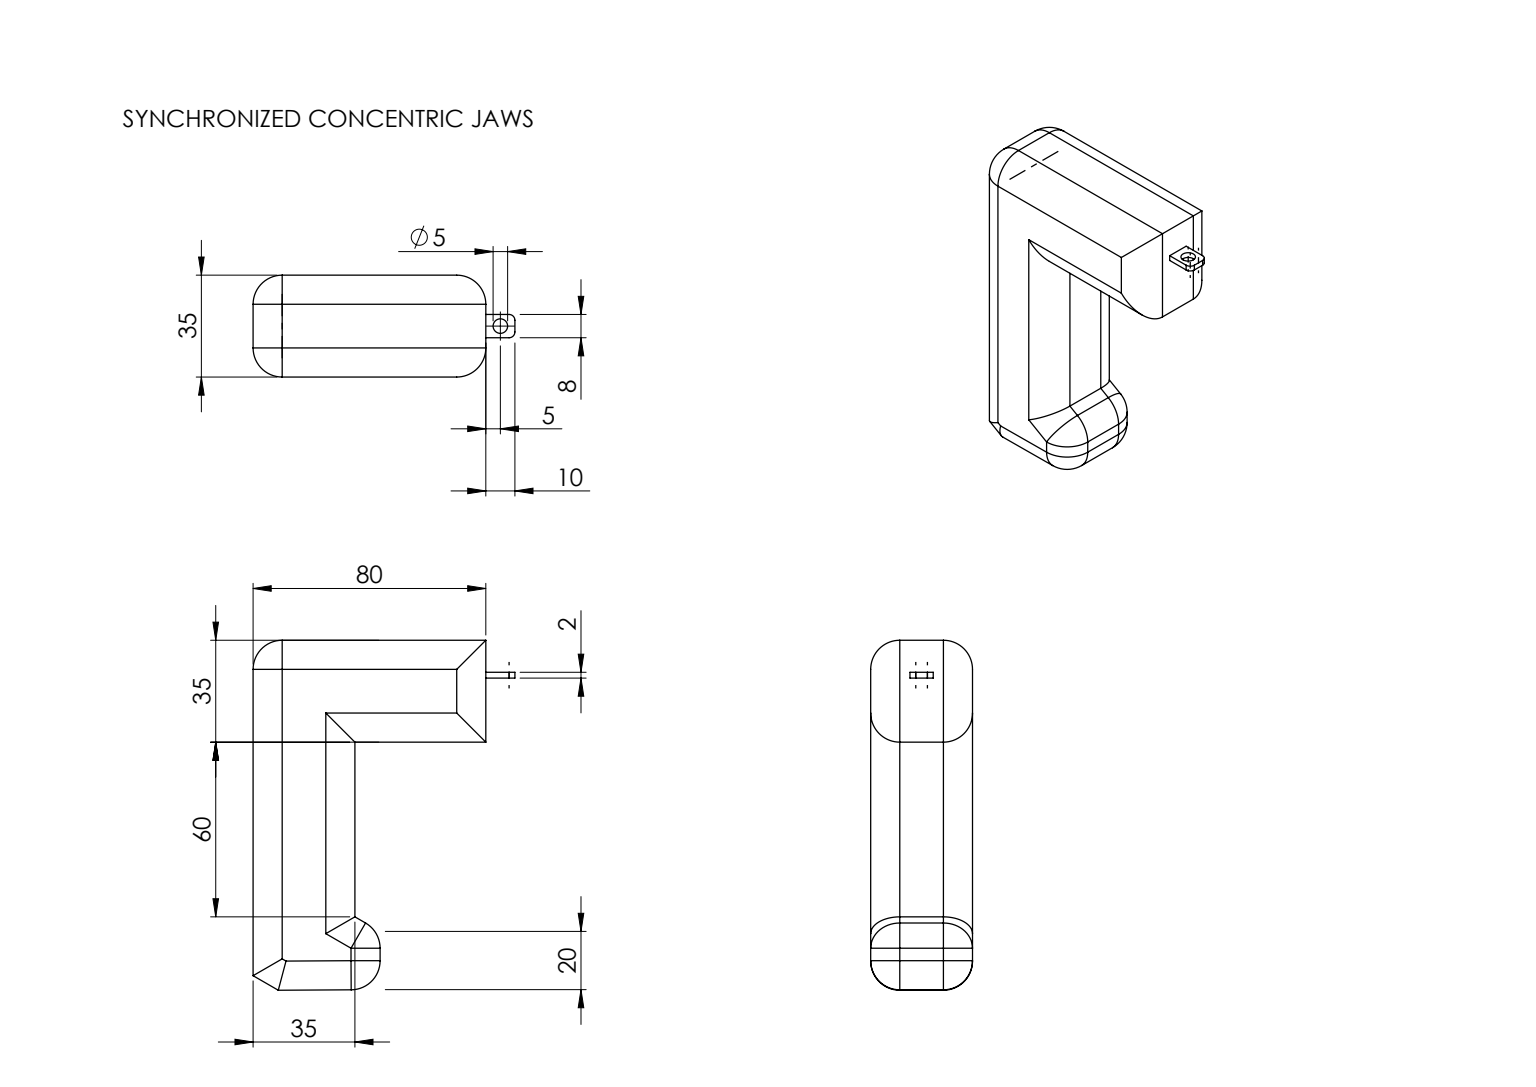
ISO-10303-21;
HEADER;
FILE_DESCRIPTION (('STEP AP214'),
    '1' );
FILE_NAME ('Synchronized Concentric Jaws.step',
    '2026-10-08T13:56:24',
    ( '' ),
    ( '' ),
    'SwSTEP 2.0',
    'SolidWorks 2026',
    '' );
FILE_SCHEMA (( 'AUTOMOTIVE_DESIGN' ));
ENDSEC;

DATA;
#2=EDGE_CURVE ( 'NONE', #5376, #11920, #8952, .T. ) ;
#20=ORIENTED_EDGE ( 'NONE', *, *, #13802, .F. ) ;
#26=ORIENTED_EDGE ( 'NONE', *, *, #11739, .T. ) ;
#47=FACE_OUTER_BOUND ( 'NONE', #13583, .T. ) ;
#72=ORIENTED_EDGE ( 'NONE', *, *, #13780, .T. ) ;
#78=DIRECTION ( 'NONE',  ( -1.000000000000000000, 0.000000000000000000, 0.000000000000000000 ) ) ;
#80=LINE ( 'NONE', #11141, #9950 ) ;
#112=DIRECTION ( 'NONE',  ( -1.925929944387236904E-30, 1.000000000000000000, -1.387778780781445676E-15 ) ) ;
#145=EDGE_CURVE ( 'NONE', #14420, #4422, #3824, .T. ) ;
#155=AXIS2_PLACEMENT_3D ( 'NONE', #3936, #13786, #7593 ) ;
#160=VECTOR ( 'NONE', #2348, 1000.000000000000000 ) ;
#188=EDGE_LOOP ( 'NONE', ( #9536, #20, #1499, #15874 ) ) ;
#190=VECTOR ( 'NONE', #3523, 1000.000000000000000 ) ;
#206=ORIENTED_EDGE ( 'NONE', *, *, #3407, .T. ) ;
#212=CARTESIAN_POINT ( 'NONE',  ( -44.99999999999999289, -11.00000000000000178, 4.000000000000831335 ) ) ;
#224=ORIENTED_EDGE ( 'NONE', *, *, #11721, .F. ) ;
#231=AXIS2_PLACEMENT_3D ( 'NONE', #4894, #14440, #11914 ) ;
#238=CARTESIAN_POINT ( 'NONE',  ( -115.0000000000000142, -3.122502256758252770E-14, 7.500000000000001776 ) ) ;
#253=CARTESIAN_POINT ( 'NONE',  ( -36.99999999999999289, -11.00000000000000178, 4.000000000000832223 ) ) ;
#283=ORIENTED_EDGE ( 'NONE', *, *, #4424, .F. ) ;
#306=ORIENTED_EDGE ( 'NONE', *, *, #14745, .F. ) ;
#310=DIRECTION ( 'NONE',  ( -1.000000000000000000, -2.775557561562892929E-15, 0.000000000000000000 ) ) ;
#317=FACE_OUTER_BOUND ( 'NONE', #13857, .T. ) ;
#319=CARTESIAN_POINT ( 'NONE',  ( -158.0560796608385488, -84.57531754730580076, 7.500000000000001776 ) ) ;
#326=ORIENTED_EDGE ( 'NONE', *, *, #10294, .F. ) ;
#344=ORIENTED_EDGE ( 'NONE', *, *, #14576, .T. ) ;
#350=CARTESIAN_POINT ( 'NONE',  ( -90.00000000000000000, -95.00000000000000000, 7.500000000000001776 ) ) ;
#373=ORIENTED_EDGE ( 'NONE', *, *, #7059, .F. ) ;
#393=EDGE_LOOP ( 'NONE', ( #15689, #8043, #13858, #8283 ) ) ;
#394=DIRECTION ( 'NONE',  ( -0.000000000000000000, -1.000000000000000000, -0.000000000000000000 ) ) ;
#396=SHAPE_REPRESENTATION ( 'Synchronized Concentric Jaws', ( #3223 ), #1155 ) ;
#443=ORIENTED_EDGE ( 'NONE', *, *, #6817, .F. ) ;
#451=ADVANCED_FACE ( 'NONE', ( #852 ), #7980, .T. ) ;
#461=ORIENTED_EDGE ( 'NONE', *, *, #7687, .F. ) ;
#466=AXIS2_PLACEMENT_3D ( 'NONE', #5707, #10643, #4493 ) ;
#472=DIRECTION ( 'NONE',  ( 0.000000000000000000, -1.000000000000000000, 0.000000000000000000 ) ) ;
#486=DIRECTION ( 'NONE',  ( -1.387778780781446464E-15, -1.000000000000000000, 1.387778780781447648E-15 ) ) ;
#525=( NAMED_UNIT ( * ) SI_UNIT ( $, .STERADIAN. ) SOLID_ANGLE_UNIT ( ) );
#546=ORIENTED_EDGE ( 'NONE', *, *, #11089, .F. ) ;
#549=FACE_OUTER_BOUND ( 'NONE', #2959, .T. ) ;
#554=FACE_OUTER_BOUND ( 'NONE', #8051, .T. ) ;
#559=LINE ( 'NONE', #10495, #3498 ) ;
#564=ORIENTED_EDGE ( 'NONE', *, *, #15075, .T. ) ;
#582=VECTOR ( 'NONE', #7048, 1000.000000000000000 ) ;
#586=EDGE_CURVE ( 'NONE', #13829, #5811, #14718, .T. ) ;
#597=DIRECTION ( 'NONE',  ( 1.000000000000000000, 1.239088197126290324E-16, -0.000000000000000000 ) ) ;
#617=CARTESIAN_POINT ( 'NONE',  ( -81.33974596215558961, -105.7735026918962404, 17.50000000000000000 ) ) ;
#619=EDGE_LOOP ( 'NONE', ( #15665, #842, #2905, #10808 ) ) ;
#630=CARTESIAN_POINT ( 'NONE',  ( -91.28042740779480368, -120.0589677227266918, -7.500000000000000000 ) ) ;
#645=AXIS2_PLACEMENT_3D ( 'NONE', #6232, #7360, #12268 ) ;
#651=LINE ( 'NONE', #15677, #14820 ) ;
#658=VERTEX_POINT ( 'NONE', #6156 ) ;
#665=CARTESIAN_POINT ( 'NONE',  ( -94.14213562373093680, -97.39146311738103634, 17.50000000000001421 ) ) ;
#677=VECTOR ( 'NONE', #5737, 1000.000000000000000 ) ;
#683=CARTESIAN_POINT ( 'NONE',  ( -44.99999999999999289, -35.00000000000000000, 17.50000000000000000 ) ) ;
#696=ORIENTED_EDGE ( 'NONE', *, *, #9480, .F. ) ;
#707=CARTESIAN_POINT ( 'NONE',  ( -99.99999999999998579, -25.00000000000000711, 17.50000000000000000 ) ) ;
#718=ORIENTED_EDGE ( 'NONE', *, *, #3664, .F. ) ;
#722=CYLINDRICAL_SURFACE ( 'NONE', #11218, 10.00000000000000000 ) ;
#757=VERTEX_POINT ( 'NONE', #7935 ) ;
#765=DIRECTION ( 'NONE',  ( -0.000000000000000000, -0.000000000000000000, -1.000000000000000000 ) ) ;
#770=EDGE_LOOP ( 'NONE', ( #1058, #1735, #5015, #1295 ) ) ;
#785=CARTESIAN_POINT ( 'NONE',  ( -114.9999999999999858, -115.2072594216369907, 17.50000000000000000 ) ) ;
#794=VERTEX_POINT ( 'NONE', #12509 ) ;
#798=DIRECTION ( 'NONE',  ( 0.4999999999999976685, 0.8660254037844399289, 0.000000000000000000 ) ) ;
#807=LINE ( 'NONE', #5727, #13340 ) ;
#811=DIRECTION ( 'NONE',  ( 1.319090325525611458E-16, 1.000000000000000000, 0.000000000000000000 ) ) ;
#820=CARTESIAN_POINT ( 'NONE',  ( -54.99999999999999289, -25.00000000000000000, 17.50000000000000000 ) ) ;
#842=ORIENTED_EDGE ( 'NONE', *, *, #8606, .F. ) ;
#845=LINE ( 'NONE', #15641, #3770 ) ;
#852=FACE_OUTER_BOUND ( 'NONE', #5733, .T. ) ;
#883=CARTESIAN_POINT ( 'NONE',  ( -39.99999999999999289, -11.00000000000000178, -2.500000000000079492 ) ) ;
#930=ORIENTED_EDGE ( 'NONE', *, *, #7501, .T. ) ;
#964=ORIENTED_EDGE ( 'NONE', *, *, #14576, .F. ) ;
#966=ORIENTED_EDGE ( 'NONE', *, *, #12050, .T. ) ;
#977=DIRECTION ( 'NONE',  ( -0.8660254037844401509, 0.4999999999999973355, -0.000000000000000000 ) ) ;
#979=EDGE_CURVE ( 'NONE', #13100, #8026, #12847, .T. ) ;
#992=ADVANCED_FACE ( 'NONE', ( #2100 ), #5909, .T. ) ;
#1013=CARTESIAN_POINT ( 'NONE',  ( -150.5560796608385203, -71.58493649053926333, -17.50000000000000000 ) ) ;
#1024=ORIENTED_EDGE ( 'NONE', *, *, #7059, .T. ) ;
#1028=FACE_BOUND ( 'NONE', #13834, .T. ) ;
#1046=DIRECTION ( 'NONE',  ( 0.9999824063907751803, 0.005931855436079011210, -0.000000000000000000 ) ) ;
#1058=ORIENTED_EDGE ( 'NONE', *, *, #12944, .T. ) ;
#1060=EDGE_CURVE ( 'NONE', #5100, #14039, #4611, .T. ) ;
#1072=EDGE_CURVE ( 'NONE', #12769, #13901, #14197, .T. ) ;
#1083=CARTESIAN_POINT ( 'NONE',  ( -111.3391301858327296, -111.5473609024183475, 17.50000000000000000 ) ) ;
#1090=CYLINDRICAL_SURFACE ( 'NONE', #14091, 10.00000000000000000 ) ;
#1114=EDGE_CURVE ( 'NONE', #794, #15817, #9839, .T. ) ;
#1117=ORIENTED_EDGE ( 'NONE', *, *, #12225, .T. ) ;
#1129=DIRECTION ( 'NONE',  ( 0.000000000000000000, -0.000000000000000000, -1.000000000000000000 ) ) ;
#1148=ORIENTED_EDGE ( 'NONE', *, *, #5739, .F. ) ;
#1155=( GEOMETRIC_REPRESENTATION_CONTEXT ( 3 ) GLOBAL_UNCERTAINTY_ASSIGNED_CONTEXT ( ( #5133 ) ) GLOBAL_UNIT_ASSIGNED_CONTEXT ( ( #12689, #7870, #525 ) ) REPRESENTATION_CONTEXT ( 'NONE', 'WORKASPACE' ) );
#1159=CARTESIAN_POINT ( 'NONE',  ( -113.6871902368262965, -110.1917077999038099, -17.50000000000000000 ) ) ;
#1170=EDGE_LOOP ( 'NONE', ( #3935, #2515, #6182 ) ) ;
#1175=AXIS2_PLACEMENT_3D ( 'NONE', #12176, #78, #12343 ) ;
#1181=EDGE_CURVE ( 'NONE', #6165, #13829, #13462, .T. ) ;
#1200=CARTESIAN_POINT ( 'NONE',  ( -81.33974596215560382, -110.0591436588189538, -7.500000000000000000 ) ) ;
#1203=DIRECTION ( 'NONE',  ( 1.000000000000000000, 0.000000000000000000, -0.000000000000000000 ) ) ;
#1226=FACE_OUTER_BOUND ( 'NONE', #7970, .T. ) ;
#1242=VECTOR ( 'NONE', #8938, 1000.000000000000000 ) ;
#1255=VECTOR ( 'NONE', #10833, 1000.000000000000000 ) ;
#1259=EDGE_CURVE ( 'NONE', #10280, #10210, #6230, .T. ) ;
#1261=EDGE_CURVE ( 'NONE', #11117, #5376, #7210, .T. ) ;
#1276=CARTESIAN_POINT ( 'NONE',  ( -55.00000000000000000, -1.734723475976807094E-15, 17.50000000000000000 ) ) ;
#1290=DIRECTION ( 'NONE',  ( 0.000000000000000000, 0.000000000000000000, -1.000000000000000000 ) ) ;
#1295=ORIENTED_EDGE ( 'NONE', *, *, #8606, .T. ) ;
#1306=DIRECTION ( 'NONE',  ( -0.8660254037844407060, 0.4999999999999965583, 0.000000000000000000 ) ) ;
#1314=ORIENTED_EDGE ( 'NONE', *, *, #10414, .F. ) ;
#1344=DIRECTION ( 'NONE',  ( 1.319090325525611458E-16, 1.000000000000000000, -0.000000000000000000 ) ) ;
#1352=DIRECTION ( 'NONE',  ( 0.000000000000000000, 1.000000000000000000, 0.000000000000000000 ) ) ;
#1360=DIRECTION ( 'NONE',  ( -0.000000000000000000, 0.000000000000000000, 1.000000000000000000 ) ) ;
#1362=FACE_OUTER_BOUND ( 'NONE', #8809, .T. ) ;
#1372=ORIENTED_EDGE ( 'NONE', *, *, #14448, .F. ) ;
#1395=AXIS2_PLACEMENT_3D ( 'NONE', #13554, #2487, #7448 ) ;
#1419=ADVANCED_FACE ( 'NONE', ( #7691 ), #1687, .F. ) ;
#1477=CYLINDRICAL_SURFACE ( 'NONE', #2817, 10.00000000000000000 ) ;
#1496=CARTESIAN_POINT ( 'NONE',  ( -49.14213562373093680, -4.142135623730950122, 17.49999999999999645 ) ) ;
#1498=DIRECTION ( 'NONE',  ( -1.000000000000000000, 1.387778780781446464E-15, 0.000000000000000000 ) ) ;
#1499=ORIENTED_EDGE ( 'NONE', *, *, #1640, .F. ) ;
#1500=DIRECTION ( 'NONE',  ( 1.982541115402065110E-16, -1.000000000000000000, 0.000000000000000000 ) ) ;
#1508=CARTESIAN_POINT ( 'NONE',  ( -91.33974596215558961, -110.0591436588189254, 7.500000000000001776 ) ) ;
#1515=FACE_OUTER_BOUND ( 'NONE', #7353, .T. ) ;
#1529=DIRECTION ( 'NONE',  ( -1.387778780781446464E-15, -1.000000000000000000, -0.000000000000000000 ) ) ;
#1530=EDGE_LOOP ( 'NONE', ( #4141, #4262 ) ) ;
#1541=LINE ( 'NONE', #13807, #12251 ) ;
#1545=ORIENTED_EDGE ( 'NONE', *, *, #13780, .F. ) ;
#1547=VERTEX_POINT ( 'NONE', #14221 ) ;
#1560=CARTESIAN_POINT ( 'NONE',  ( -114.4056415360013688, -110.1959696241292335, -17.50000000000000000 ) ) ;
#1570=CARTESIAN_POINT ( 'NONE',  ( -55.00000000000000000, -10.00000000000000178, 17.50000000000000000 ) ) ;
#1587=CARTESIAN_POINT ( 'NONE',  ( -44.99999999999999289, -11.00000000000000178, -3.999999999999170885 ) ) ;
#1589=CARTESIAN_POINT ( 'NONE',  ( -49.14213562373093680, -30.85786437626904899, -17.49999999999999645 ) ) ;
#1597=VERTEX_POINT ( 'NONE', #11053 ) ;
#1610=EDGE_CURVE ( 'NONE', #10210, #14193, #2463, .T. ) ;
#1614=ORIENTED_EDGE ( 'NONE', *, *, #11960, .F. ) ;
#1640=EDGE_CURVE ( 'NONE', #15020, #3371, #4274, .T. ) ;
#1649=CARTESIAN_POINT ( 'NONE',  ( -116.3391301858327296, -120.2076149402627294, 7.500000000000001776 ) ) ;
#1652=DIRECTION ( 'NONE',  ( 0.000000000000000000, 0.000000000000000000, 1.000000000000000000 ) ) ;
#1684=EDGE_CURVE ( 'NONE', #4500, #5972, #13528, .T. ) ;
#1687=CYLINDRICAL_SURFACE ( 'NONE', #11678, 2.500000000000909495 ) ;
#1702=ORIENTED_EDGE ( 'NONE', *, *, #2061, .F. ) ;
#1727=DIRECTION ( 'NONE',  ( -0.000000000000000000, -1.000000000000000000, -0.000000000000000000 ) ) ;
#1734=DIRECTION ( 'NONE',  ( -1.982541115402065110E-16, 1.000000000000000000, 0.000000000000000000 ) ) ;
#1735=ORIENTED_EDGE ( 'NONE', *, *, #4357, .T. ) ;
#1736=ORIENTED_EDGE ( 'NONE', *, *, #7501, .F. ) ;
#1743=CIRCLE ( 'NONE', #3807, 9.999999999999994671 ) ;
#1763=CARTESIAN_POINT ( 'NONE',  ( -91.33974596215560382, -110.0591436588189396, -17.50000000000000000 ) ) ;
#1815=ORIENTED_EDGE ( 'NONE', *, *, #11551, .T. ) ;
#1858=CARTESIAN_POINT ( 'NONE',  ( -89.99999999999997158, -95.00000000000001421, 13.35786437626905965 ) ) ;
#1884=CYLINDRICAL_SURFACE ( 'NONE', #12589, 2.000000000000000888 ) ;
#1886=VERTEX_POINT ( 'NONE', #9424 ) ;
#1893=DIRECTION ( 'NONE',  ( -0.000000000000000000, -1.000000000000000000, -0.000000000000000000 ) ) ;
#1905=( BOUNDED_CURVE ( )  B_SPLINE_CURVE ( 3, ( #6211, #13529, #3857, #9909 ),
 .UNSPECIFIED., .F., .F. ) 
 B_SPLINE_CURVE_WITH_KNOTS ( ( 4, 4 ),
 ( 1.570796326794895226, 3.141592653589793116 ),
 .UNSPECIFIED. ) 
 CURVE ( )  GEOMETRIC_REPRESENTATION_ITEM ( )  RATIONAL_B_SPLINE_CURVE ( ( 1.000000000000000000, 0.8047378541243646044, 0.8047378541243646044, 1.000000000000000000 ) ) 
 REPRESENTATION_ITEM ( '' )  );
#1936=ORIENTED_EDGE ( 'NONE', *, *, #15075, .F. ) ;
#1959=CARTESIAN_POINT ( 'NONE',  ( -115.0000000000000142, -10.00000000000000888, 7.500000000000001776 ) ) ;
#1995=EDGE_CURVE ( 'NONE', #14464, #5100, #13505, .T. ) ;
#2019=VECTOR ( 'NONE', #7235, 1000.000000000000000 ) ;
#2023=CARTESIAN_POINT ( 'NONE',  ( -45.00000000000000000, 0.000000000000000000, 17.50000000000000000 ) ) ;
#2033=VECTOR ( 'NONE', #10246, 1000.000000000000000 ) ;
#2042=EDGE_CURVE ( 'NONE', #15020, #15896, #12067, .T. ) ;
#2055=CARTESIAN_POINT ( 'NONE',  ( -114.4056415360013688, -110.1959696241292335, 7.500000000000001776 ) ) ;
#2058=DIRECTION ( 'NONE',  ( 0.000000000000000000, 0.000000000000000000, -1.000000000000000000 ) ) ;
#2060=CARTESIAN_POINT ( 'NONE',  ( -116.3391301858327296, -120.2076149402627294, -7.500000000000000000 ) ) ;
#2061=EDGE_CURVE ( 'NONE', #14193, #7180, #15739, .T. ) ;
#2066=LINE ( 'NONE', #785, #13594 ) ;
#2084=CARTESIAN_POINT ( 'NONE',  ( -114.9999999999999858, -109.4337567297407219, -17.50000000000000000 ) ) ;
#2099=CARTESIAN_POINT ( 'NONE',  ( -44.99999999999999289, -35.00000000000000000, 17.50000000000000000 ) ) ;
#2100=FACE_OUTER_BOUND ( 'NONE', #15094, .T. ) ;
#2125=ORIENTED_EDGE ( 'NONE', *, *, #10428, .T. ) ;
#2133=AXIS2_PLACEMENT_3D ( 'NONE', #13779, #2714, #472 ) ;
#2153=PRODUCT_DEFINITION ( 'UNKNOWN', '', #5085, #2371 ) ;
#2155=LINE ( 'NONE', #12005, #190 ) ;
#2212=DIRECTION ( 'NONE',  ( 0.000000000000000000, 1.000000000000000000, 0.000000000000000000 ) ) ;
#2224=CIRCLE ( 'NONE', #11263, 2.500000000000909495 ) ;
#2256=SPHERICAL_SURFACE ( 'NONE', #9506, 10.00000000000000000 ) ;
#2258=AXIS2_PLACEMENT_3D ( 'NONE', #10852, #15792, #7303 ) ;
#2293=EDGE_LOOP ( 'NONE', ( #12874, #3623, #1545, #4562 ) ) ;
#2308=AXIS2_PLACEMENT_3D ( 'NONE', #7872, #8843, #13748 ) ;
#2311=EDGE_LOOP ( 'NONE', ( #5185, #10664, #326, #13860 ) ) ;
#2314=CARTESIAN_POINT ( 'NONE',  ( -115.0000000000000142, -10.00000000000000888, 7.500000000000001776 ) ) ;
#2315=CARTESIAN_POINT ( 'NONE',  ( -114.9999999999999858, -109.4337567297407219, -17.50000000000000000 ) ) ;
#2327=ORIENTED_EDGE ( 'NONE', *, *, #13355, .F. ) ;
#2332=ORIENTED_EDGE ( 'NONE', *, *, #12839, .T. ) ;
#2334=EDGE_CURVE ( 'NONE', #3131, #15817, #13089, .T. ) ;
#2345=FACE_BOUND ( 'NONE', #1530, .T. ) ;
#2348=DIRECTION ( 'NONE',  ( -6.938893903907228378E-16, -1.000000000000000000, 0.000000000000000000 ) ) ;
#2370=DIRECTION ( 'NONE',  ( -1.982541115402065110E-16, 1.000000000000000000, 0.000000000000000000 ) ) ;
#2371=PRODUCT_DEFINITION_CONTEXT ( 'detailed design', #7449, 'design' ) ;
#2385=DIRECTION ( 'NONE',  ( 1.982541115402065110E-16, -1.000000000000000000, 0.000000000000000000 ) ) ;
#2396=ORIENTED_EDGE ( 'NONE', *, *, #12301, .F. ) ;
#2413=ORIENTED_EDGE ( 'NONE', *, *, #14745, .T. ) ;
#2414=EDGE_CURVE ( 'NONE', #13901, #3131, #8820, .T. ) ;
#2441=FACE_OUTER_BOUND ( 'NONE', #3474, .T. ) ;
#2442=CARTESIAN_POINT ( 'NONE',  ( -45.00000000000000000, 0.000000000000000000, -7.500000000000000000 ) ) ;
#2447=ADVANCED_FACE ( 'NONE', ( #4855 ), #9781, .T. ) ;
#2463=LINE ( 'NONE', #12241, #4705 ) ;
#2466=DIRECTION ( 'NONE',  ( -1.000000000000000000, 0.000000000000000000, 0.000000000000000000 ) ) ;
#2485=CARTESIAN_POINT ( 'NONE',  ( -116.3391301858327296, -120.2076149402627294, -7.500000000000000000 ) ) ;
#2487=DIRECTION ( 'NONE',  ( -1.319090325525611458E-16, -1.000000000000000000, 0.000000000000000000 ) ) ;
#2491=ADVANCED_FACE ( 'NONE', ( #3709 ), #8656, .T. ) ;
#2496=CARTESIAN_POINT ( 'NONE',  ( -94.14213562373093680, -30.85786437626905965, 17.50000000000000000 ) ) ;
#2507=DIRECTION ( 'NONE',  ( 0.000000000000000000, 0.000000000000000000, 1.000000000000000000 ) ) ;
#2515=ORIENTED_EDGE ( 'NONE', *, *, #8358, .T. ) ;
#2520=ADVANCED_FACE ( 'NONE', ( #1362 ), #15037, .T. ) ;
#2525=PLANE ( 'NONE',  #11792 ) ;
#2528=DIRECTION ( 'NONE',  ( -1.982541115402065110E-16, 1.000000000000000000, 0.000000000000000000 ) ) ;
#2549=CARTESIAN_POINT ( 'NONE',  ( -34.99999999999999289, -11.00000000000000178, -1.999999999999170441 ) ) ;
#2555=CARTESIAN_POINT ( 'NONE',  ( -114.9999999999999716, -10.00000000000000888, -17.50000000000000000 ) ) ;
#2567=DIRECTION ( 'NONE',  ( -0.000000000000000000, -0.000000000000000000, -1.000000000000000000 ) ) ;
#2581=ORIENTED_EDGE ( 'NONE', *, *, #1261, .T. ) ;
#2589=EDGE_CURVE ( 'NONE', #14039, #7722, #9908, .T. ) ;
#2592=PRODUCT_CONTEXT ( 'NONE', #12774, 'mechanical' ) ;
#2594=DIRECTION ( 'NONE',  ( 1.000000000000000000, 0.000000000000000000, -0.000000000000000000 ) ) ;
#2613=DIRECTION ( 'NONE',  ( 0.9999824063907751803, 0.005931855436079011210, -0.000000000000000000 ) ) ;
#2630=CARTESIAN_POINT ( 'NONE',  ( -44.99999999999999289, -11.00000000000000178, -3.999999999999170885 ) ) ;
#2632=DIRECTION ( 'NONE',  ( 1.982541115402065110E-16, -1.000000000000000000, -0.000000000000000000 ) ) ;
#2639=ORIENTED_EDGE ( 'NONE', *, *, #2061, .T. ) ;
#2712=LINE ( 'NONE', #12405, #12601 ) ;
#2714=DIRECTION ( 'NONE',  ( -1.000000000000000000, -1.239088197126290324E-16, 0.000000000000000000 ) ) ;
#2735=CIRCLE ( 'NONE', #5835, 10.00000000000000533 ) ;
#2750=CLOSED_SHELL ( 'NONE', ( #11744, #13481, #12892, #14008, #15031, #2796, #9089, #7588, #7423, #3759, #9766, #4823, #3876, #5608, #14695, #5039, #451, #4544, #9312, #9707, #1419, #5923, #8038, #10795, #5536, #15578, #3060, #10962, #9054, #2447, #6622, #10571, #13675, #10631, #9499, #2491, #3085, #3960, #4359, #13345, #10515, #2520, #14408, #13001, #10591, #3464, #992 ) ) ;
#2752=EDGE_CURVE ( 'NONE', #7410, #14039, #651, .T. ) ;
#2753=AXIS2_PLACEMENT_3D ( 'NONE', #9504, #2212, #14892 ) ;
#2761=SPHERICAL_SURFACE ( 'NONE', #5838, 10.00000000000000000 ) ;
#2762=ORIENTED_EDGE ( 'NONE', *, *, #2, .T. ) ;
#2789=VERTEX_POINT ( 'NONE', #15521 ) ;
#2790=VERTEX_POINT ( 'NONE', #3220 ) ;
#2796=ADVANCED_FACE ( 'NONE', ( #8169 ), #13071, .F. ) ;
#2800=DIRECTION ( 'NONE',  ( -0.4999999999999965028, -0.8660254037844407060, 0.000000000000000000 ) ) ;
#2808=VERTEX_POINT ( 'NONE', #883 ) ;
#2817=AXIS2_PLACEMENT_3D ( 'NONE', #3973, #597, #10376 ) ;
#2823=DIRECTION ( 'NONE',  ( 1.000000000000000000, 1.239088197126290324E-16, -0.000000000000000000 ) ) ;
#2859=LINE ( 'NONE', #1649, #5065 ) ;
#2865=EDGE_CURVE ( 'NONE', #5376, #13100, #13225, .T. ) ;
#2905=ORIENTED_EDGE ( 'NONE', *, *, #7446, .F. ) ;
#2906=EDGE_LOOP ( 'NONE', ( #14722, #12535, #546, #461 ) ) ;
#2909=ORIENTED_EDGE ( 'NONE', *, *, #9480, .T. ) ;
#2920=ORIENTED_EDGE ( 'NONE', *, *, #4424, .T. ) ;
#2932=CARTESIAN_POINT ( 'NONE',  ( -36.99999999999999289, -11.00000000000000178, -1.999999999999170885 ) ) ;
#2935=CYLINDRICAL_SURFACE ( 'NONE', #15701, 10.00000000000000178 ) ;
#2948=EDGE_CURVE ( 'NONE', #4422, #13155, #14768, .T. ) ;
#2959=EDGE_LOOP ( 'NONE', ( #4836, #7640, #283, #1936 ) ) ;
#2962=ORIENTED_EDGE ( 'NONE', *, *, #4129, .T. ) ;
#2965=ORIENTED_EDGE ( 'NONE', *, *, #12944, .F. ) ;
#2978=DIRECTION ( 'NONE',  ( 0.000000000000000000, 0.000000000000000000, 1.000000000000000000 ) ) ;
#3033=EDGE_CURVE ( 'NONE', #10280, #14464, #11078, .T. ) ;
#3060=ADVANCED_FACE ( 'NONE', ( #554 ), #6696, .T. ) ;
#3085=ADVANCED_FACE ( 'NONE', ( #9119 ), #11367, .T. ) ;
#3091=DIRECTION ( 'NONE',  ( 6.938893903907228378E-16, 1.000000000000000000, -0.000000000000000000 ) ) ;
#3101=CARTESIAN_POINT ( 'NONE',  ( -34.99999999999999289, -13.00000000000000178, -1.999999999999170441 ) ) ;
#3105=VECTOR ( 'NONE', #11656, 1000.000000000000000 ) ;
#3116=DIRECTION ( 'NONE',  ( -1.000000000000000000, 1.734723475976808080E-16, 0.000000000000000000 ) ) ;
#3127=DIRECTION ( 'NONE',  ( 0.000000000000000000, 0.000000000000000000, -1.000000000000000000 ) ) ;
#3131=VERTEX_POINT ( 'NONE', #707 ) ;
#3164=EDGE_CURVE ( 'NONE', #10935, #4422, #7069, .T. ) ;
#3172=SPHERICAL_SURFACE ( 'NONE', #8273, 10.00000000000000000 ) ;
#3195=CARTESIAN_POINT ( 'NONE',  ( -124.9999999999999716, -10.00000000000001066, 7.500000000000001776 ) ) ;
#3201=FACE_OUTER_BOUND ( 'NONE', #15843, .T. ) ;
#3220=CARTESIAN_POINT ( 'NONE',  ( -34.99999999999999289, -11.00000000000000178, -1.999999999999170441 ) ) ;
#3223=AXIS2_PLACEMENT_3D ( 'NONE', #11897, #11972, #4638 ) ;
#3305=DIRECTION ( 'NONE',  ( 0.4999999999999973355, 0.8660254037844402619, -0.000000000000000000 ) ) ;
#3331=CARTESIAN_POINT ( 'NONE',  ( -91.33974596215558961, -110.0591436588189254, 17.50000000000000000 ) ) ;
#3349=CARTESIAN_POINT ( 'NONE',  ( -113.6871902368263250, -110.1917077999037957, 17.50000000000000000 ) ) ;
#3371=VERTEX_POINT ( 'NONE', #9650 ) ;
#3386=MANIFOLD_SOLID_BREP ( 'Fillet1', #2750 ) ;
#3399=FACE_OUTER_BOUND ( 'NONE', #15186, .T. ) ;
#3407=EDGE_CURVE ( 'NONE', #8136, #14464, #7485, .T. ) ;
#3417=ORIENTED_EDGE ( 'NONE', *, *, #15234, .T. ) ;
#3425=EDGE_CURVE ( 'NONE', #9981, #757, #15430, .T. ) ;
#3434=ORIENTED_EDGE ( 'NONE', *, *, #3164, .T. ) ;
#3438=ORIENTED_EDGE ( 'NONE', *, *, #6306, .F. ) ;
#3446=FACE_OUTER_BOUND ( 'NONE', #1170, .T. ) ;
#3454=DIRECTION ( 'NONE',  ( 0.8660254037844405950, -0.4999999999999965028, -0.000000000000000000 ) ) ;
#3464=ADVANCED_FACE ( 'NONE', ( #4071 ), #11500, .T. ) ;
#3474=EDGE_LOOP ( 'NONE', ( #14614, #12377, #2125, #4222, #11847, #9762, #6762, #14706, #14265 ) ) ;
#3476=VERTEX_POINT ( 'NONE', #12629 ) ;
#3477=CARTESIAN_POINT ( 'NONE',  ( -91.33974596215551855, -10.00000000000002487, -17.50000000000000000 ) ) ;
#3490=LINE ( 'NONE', #4713, #2019 ) ;
#3495=ORIENTED_EDGE ( 'NONE', *, *, #7519, .T. ) ;
#3498=VECTOR ( 'NONE', #4013, 1000.000000000000000 ) ;
#3515=EDGE_CURVE ( 'NONE', #15896, #5616, #5137, .T. ) ;
#3522=CIRCLE ( 'NONE', #2753, 2.500000000000909495 ) ;
#3523=DIRECTION ( 'NONE',  ( -0.000000000000000000, -0.000000000000000000, -1.000000000000000000 ) ) ;
#3534=CARTESIAN_POINT ( 'NONE',  ( -39.99999999999999289, -13.00000000000000178, -2.500000000000079492 ) ) ;
#3545=VECTOR ( 'NONE', #2823, 1000.000000000000000 ) ;
#3547=DIRECTION ( 'NONE',  ( 1.000000000000000000, 0.000000000000000000, 0.000000000000000000 ) ) ;
#3562=EDGE_CURVE ( 'NONE', #8889, #3476, #6992, .T. ) ;
#3590=DIRECTION ( 'NONE',  ( 0.000000000000000000, 0.000000000000000000, -1.000000000000000000 ) ) ;
#3623=ORIENTED_EDGE ( 'NONE', *, *, #6577, .F. ) ;
#3648=EDGE_CURVE ( 'NONE', #658, #7722, #9332, .T. ) ;
#3659=CARTESIAN_POINT ( 'NONE',  ( -91.33974596215560382, -110.0591436588189396, 7.500000000000001776 ) ) ;
#3664=EDGE_CURVE ( 'NONE', #9005, #13100, #13108, .T. ) ;
#3690=DIRECTION ( 'NONE',  ( -1.000000000000000000, -0.000000000000000000, -0.000000000000000000 ) ) ;
#3709=FACE_OUTER_BOUND ( 'NONE', #12234, .T. ) ;
#3717=AXIS2_PLACEMENT_3D ( 'NONE', #10186, #2978, #7932 ) ;
#3723=EDGE_LOOP ( 'NONE', ( #14344, #10607, #10726, #10650 ) ) ;
#3736=DIRECTION ( 'NONE',  ( -0.005931855436079598413, 0.9999824063907751803, 0.000000000000000000 ) ) ;
#3746=CYLINDRICAL_SURFACE ( 'NONE', #4364, 10.00000000000000178 ) ;
#3752=CARTESIAN_POINT ( 'NONE',  ( -86.33974596215563224, -97.11324865405184426, -7.500000000000000000 ) ) ;
#3756=ORIENTED_EDGE ( 'NONE', *, *, #2865, .F. ) ;
#3757=EDGE_LOOP ( 'NONE', ( #11136, #9700, #964, #2413 ) ) ;
#3759=ADVANCED_FACE ( 'NONE', ( #9632 ), #13182, .F. ) ;
#3770=VECTOR ( 'NONE', #10560, 1000.000000000000000 ) ;
#3802=ORIENTED_EDGE ( 'NONE', *, *, #15234, .F. ) ;
#3804=CARTESIAN_POINT ( 'NONE',  ( -90.00000000000000000, -35.00000000000000711, 7.500000000000001776 ) ) ;
#3807=AXIS2_PLACEMENT_3D ( 'NONE', #10614, #6741, #11641 ) ;
#3817=CYLINDRICAL_SURFACE ( 'NONE', #6946, 9.999999999999992895 ) ;
#3818=ORIENTED_EDGE ( 'NONE', *, *, #12542, .F. ) ;
#3824=LINE ( 'NONE', #8927, #13058 ) ;
#3857=CARTESIAN_POINT ( 'NONE',  ( -116.3391301858327438, -120.2076149402627152, 13.35786437626905965 ) ) ;
#3876=ADVANCED_FACE ( 'NONE', ( #5026 ), #9956, .F. ) ;
#3913=ORIENTED_EDGE ( 'NONE', *, *, #4216, .F. ) ;
#3931=VECTOR ( 'NONE', #7336, 1000.000000000000000 ) ;
#3935=ORIENTED_EDGE ( 'NONE', *, *, #11944, .T. ) ;
#3936=CARTESIAN_POINT ( 'NONE',  ( -36.99999999999999289, -11.00000000000000178, -1.999999999999170885 ) ) ;
#3951=AXIS2_PLACEMENT_3D ( 'NONE', #319, #11443, #5229 ) ;
#3957=ORIENTED_EDGE ( 'NONE', *, *, #2865, .T. ) ;
#3960=ADVANCED_FACE ( 'NONE', ( #10124 ), #2761, .T. ) ;
#3973=CARTESIAN_POINT ( 'NONE',  ( -115.0000000000000142, -10.00000000000000888, 7.500000000000001776 ) ) ;
#3978=AXIS2_PLACEMENT_3D ( 'NONE', #2023, #5742, #9315 ) ;
#3983=VECTOR ( 'NONE', #1727, 1000.000000000000000 ) ;
#3998=STYLED_ITEM ( 'NONE', ( #4391 ), #6973 ) ;
#4013=DIRECTION ( 'NONE',  ( -0.000000000000000000, -1.000000000000000000, -0.000000000000000000 ) ) ;
#4054=DIRECTION ( 'NONE',  ( 0.000000000000000000, -1.000000000000000000, -2.775557561562892929E-15 ) ) ;
#4071=FACE_OUTER_BOUND ( 'NONE', #6484, .T. ) ;
#4073=LINE ( 'NONE', #13763, #3983 ) ;
#4085=CARTESIAN_POINT ( 'NONE',  ( -45.00000000000000000, 0.000000000000000000, -7.500000000000000000 ) ) ;
#4088=( GEOMETRIC_REPRESENTATION_CONTEXT ( 3 ) GLOBAL_UNCERTAINTY_ASSIGNED_CONTEXT ( ( #9358 ) ) GLOBAL_UNIT_ASSIGNED_CONTEXT ( ( #13509, #7319, #12307 ) ) REPRESENTATION_CONTEXT ( 'NONE', 'WORKASPACE' ) );
#4109=EDGE_CURVE ( 'NONE', #11530, #15795, #2859, .T. ) ;
#4129=EDGE_CURVE ( 'NONE', #8026, #6165, #9491, .T. ) ;
#4141=ORIENTED_EDGE ( 'NONE', *, *, #4746, .T. ) ;
#4146=DIRECTION ( 'NONE',  ( 1.000000000000000000, 1.734723475976808080E-16, 0.000000000000000000 ) ) ;
#4206=ORIENTED_EDGE ( 'NONE', *, *, #9325, .T. ) ;
#4216=EDGE_CURVE ( 'NONE', #5811, #6058, #8132, .T. ) ;
#4217=ORIENTED_EDGE ( 'NONE', *, *, #1259, .T. ) ;
#4220=DIRECTION ( 'NONE',  ( -0.9999824063907751803, -0.005931855436079011210, 0.000000000000000000 ) ) ;
#4222=ORIENTED_EDGE ( 'NONE', *, *, #11352, .T. ) ;
#4245=DIRECTION ( 'NONE',  ( 0.8660254037844407060, -0.4999999999999965583, 0.000000000000000000 ) ) ;
#4262=ORIENTED_EDGE ( 'NONE', *, *, #10365, .T. ) ;
#4274=( BOUNDED_CURVE ( )  B_SPLINE_CURVE ( 3, ( #10885, #9832, #14765, #5965 ),
 .UNSPECIFIED., .F., .F. ) 
 B_SPLINE_CURVE_WITH_KNOTS ( ( 4, 4 ),
 ( 1.570796326794898334, 3.141592653589793116 ),
 .UNSPECIFIED. ) 
 CURVE ( )  GEOMETRIC_REPRESENTATION_ITEM ( )  RATIONAL_B_SPLINE_CURVE ( ( 1.000000000000000000, 0.8047378541243654926, 0.8047378541243654926, 1.000000000000000000 ) ) 
 REPRESENTATION_ITEM ( '' )  );
#4302=DIRECTION ( 'NONE',  ( -1.000000000000000000, -1.541976423090495140E-16, 0.000000000000000000 ) ) ;
#4305=( NAMED_UNIT ( * ) PLANE_ANGLE_UNIT ( ) SI_UNIT ( $, .RADIAN. ) );
#4312=EDGE_CURVE ( 'NONE', #11044, #8136, #2155, .T. ) ;
#4322=PLANE ( 'NONE',  #14068 ) ;
#4341=DIRECTION ( 'NONE',  ( -6.938893903907228378E-16, -1.000000000000000000, 0.000000000000000000 ) ) ;
#4344=CYLINDRICAL_SURFACE ( 'NONE', #14407, 10.00000000000000000 ) ;
#4357=EDGE_CURVE ( 'NONE', #11193, #11117, #6040, .T. ) ;
#4359=ADVANCED_FACE ( 'NONE', ( #3446 ), #8400, .T. ) ;
#4364=AXIS2_PLACEMENT_3D ( 'NONE', #13597, #2528, #6266 ) ;
#4380=PLANE ( 'NONE',  #3978 ) ;
#4391=PRESENTATION_STYLE_ASSIGNMENT (( #14248 ) ) ;
#4393=FACE_OUTER_BOUND ( 'NONE', #5894, .T. ) ;
#4402=ORIENTED_EDGE ( 'NONE', *, *, #8108, .F. ) ;
#4405=DIRECTION ( 'NONE',  ( -1.000000000000000000, -1.541976423090495140E-16, -0.000000000000000000 ) ) ;
#4422=VERTEX_POINT ( 'NONE', #7420 ) ;
#4424=EDGE_CURVE ( 'NONE', #13829, #1597, #5343, .T. ) ;
#4430=DIRECTION ( 'NONE',  ( 1.000000000000000000, 1.239088197126290324E-16, -0.000000000000000000 ) ) ;
#4487=CYLINDRICAL_SURFACE ( 'NONE', #12754, 10.00000000000000000 ) ;
#4493=DIRECTION ( 'NONE',  ( 0.000000000000000000, 0.000000000000000000, -1.000000000000000000 ) ) ;
#4500=VERTEX_POINT ( 'NONE', #2630 ) ;
#4529=DIRECTION ( 'NONE',  ( -1.000000000000000000, 0.000000000000000000, 0.000000000000000000 ) ) ;
#4535=CARTESIAN_POINT ( 'NONE',  ( -36.99999999999999289, -11.00000000000000178, -3.999999999999170885 ) ) ;
#4539=( LENGTH_UNIT ( ) NAMED_UNIT ( * ) SI_UNIT ( .MILLI., .METRE. ) );
#4544=ADVANCED_FACE ( 'NONE', ( #6603 ), #13616, .F. ) ;
#4562=ORIENTED_EDGE ( 'NONE', *, *, #4357, .F. ) ;
#4599=CARTESIAN_POINT ( 'NONE',  ( -90.00000000000000000, -95.00000000000000000, -7.500000000000000000 ) ) ;
#4610=FACE_OUTER_BOUND ( 'NONE', #8642, .T. ) ;
#4611=LINE ( 'NONE', #8275, #9365 ) ;
#4624=ORIENTED_EDGE ( 'NONE', *, *, #145, .T. ) ;
#4637=CARTESIAN_POINT ( 'NONE',  ( -36.99999999999999289, -13.00000000000000178, 4.000000000000832223 ) ) ;
#4638=DIRECTION ( 'NONE',  ( 1.000000000000000000, 0.000000000000000000, 0.000000000000000000 ) ) ;
#4675=CARTESIAN_POINT ( 'NONE',  ( -81.33974596215556119, -99.99999999999998579, 7.500000000000001776 ) ) ;
#4676=ORIENTED_EDGE ( 'NONE', *, *, #6671, .F. ) ;
#4684=PLANE ( 'NONE',  #7411 ) ;
#4691=FACE_OUTER_BOUND ( 'NONE', #13953, .T. ) ;
#4692=LINE ( 'NONE', #14552, #8468 ) ;
#4705=VECTOR ( 'NONE', #8714, 1000.000000000000000 ) ;
#4713=CARTESIAN_POINT ( 'NONE',  ( -81.33974596215560382, -119.9999999999999716, 7.500000000000001776 ) ) ;
#4714=ORIENTED_EDGE ( 'NONE', *, *, #11944, .F. ) ;
#4715=FACE_OUTER_BOUND ( 'NONE', #188, .T. ) ;
#4742=CARTESIAN_POINT ( 'NONE',  ( -120.8578643762690348, -112.8157963042559970, -17.50000000000000000 ) ) ;
#4746=EDGE_CURVE ( 'NONE', #14971, #3476, #3522, .T. ) ;
#4756=ORIENTED_EDGE ( 'NONE', *, *, #11111, .T. ) ;
#4766=DIRECTION ( 'NONE',  ( -1.000000000000000000, -1.541976423090495140E-16, 0.000000000000000000 ) ) ;
#4773=AXIS2_PLACEMENT_3D ( 'NONE', #6841, #11748, #3590 ) ;
#4779=ORIENTED_EDGE ( 'NONE', *, *, #3033, .T. ) ;
#4780=CARTESIAN_POINT ( 'NONE',  ( -99.99999999999998579, -25.00000000000000711, 17.50000000000000000 ) ) ;
#4797=SPHERICAL_SURFACE ( 'NONE', #9295, 10.00000000000000000 ) ;
#4811=SURFACE_STYLE_USAGE ( .BOTH. , #13363 ) ;
#4812=AXIS2_PLACEMENT_3D ( 'NONE', #8675, #2507, #2594 ) ;
#4817=VERTEX_POINT ( 'NONE', #1159 ) ;
#4823=ADVANCED_FACE ( 'NONE', ( #2441 ), #13429, .T. ) ;
#4836=ORIENTED_EDGE ( 'NONE', *, *, #1072, .T. ) ;
#4855=FACE_OUTER_BOUND ( 'NONE', #2311, .T. ) ;
#4883=EDGE_LOOP ( 'NONE', ( #8058, #11186, #2909, #9567 ) ) ;
#4894=CARTESIAN_POINT ( 'NONE',  ( -116.3391301858327296, -120.2076149402627294, 17.50000000000000000 ) ) ;
#4924=LINE ( 'NONE', #11072, #8137 ) ;
#4926=LINE ( 'NONE', #6150, #11051 ) ;
#4949=CARTESIAN_POINT ( 'NONE',  ( -94.99999999999995737, -103.6602540378443962, -7.500000000000000000 ) ) ;
#4953=FACE_OUTER_BOUND ( 'NONE', #10077, .T. ) ;
#4961=UNCERTAINTY_MEASURE_WITH_UNIT (LENGTH_MEASURE( 1.000000000000000082E-05 ), #4539, 'distance_accuracy_value', 'NONE');
#4998=DIRECTION ( 'NONE',  ( -0.8660254037844405950, 0.4999999999999965028, 0.000000000000000000 ) ) ;
#5015=ORIENTED_EDGE ( 'NONE', *, *, #9686, .F. ) ;
#5026=FACE_OUTER_BOUND ( 'NONE', #7020, .T. ) ;
#5034=DIRECTION ( 'NONE',  ( 1.000000000000000000, 0.000000000000000000, -1.387778780781446464E-15 ) ) ;
#5039=ADVANCED_FACE ( 'NONE', ( #13844 ), #2525, .F. ) ;
#5048=CARTESIAN_POINT ( 'NONE',  ( -81.39906451651640396, -110.0001759360922051, 17.50000000000000000 ) ) ;
#5061=VECTOR ( 'NONE', #4430, 1000.000000000000000 ) ;
#5065=VECTOR ( 'NONE', #11504, 1000.000000000000000 ) ;
#5085=PRODUCT_DEFINITION_FORMATION_WITH_SPECIFIED_SOURCE ( 'ANY', '', #9518, .NOT_KNOWN. ) ;
#5095=CARTESIAN_POINT ( 'NONE',  ( -86.33974596215563224, -97.11324865405184426, 17.50000000000000000 ) ) ;
#5100=VERTEX_POINT ( 'NONE', #7646 ) ;
#5128=DIRECTION ( 'NONE',  ( -0.000000000000000000, -0.000000000000000000, -1.000000000000000000 ) ) ;
#5133=UNCERTAINTY_MEASURE_WITH_UNIT (LENGTH_MEASURE( 1.000000000000000082E-05 ), #12689, 'distance_accuracy_value', 'NONE');
#5137=LINE ( 'NONE', #5048, #15336 ) ;
#5145=CARTESIAN_POINT ( 'NONE',  ( -44.99999999999999289, -25.00000000000000000, -7.500000000000000000 ) ) ;
#5164=EDGE_LOOP ( 'NONE', ( #12135, #5201, #5523, #5871 ) ) ;
#5185=ORIENTED_EDGE ( 'NONE', *, *, #12542, .T. ) ;
#5198=FILL_AREA_STYLE_COLOUR ( '', #5560 ) ;
#5199=ORIENTED_EDGE ( 'NONE', *, *, #12225, .F. ) ;
#5201=ORIENTED_EDGE ( 'NONE', *, *, #14506, .F. ) ;
#5215=LINE ( 'NONE', #12555, #7911 ) ;
#5218=( BOUNDED_CURVE ( )  B_SPLINE_CURVE ( 3, ( #11904, #13121, #9797, #9500 ),
 .UNSPECIFIED., .F., .F. ) 
 B_SPLINE_CURVE_WITH_KNOTS ( ( 4, 4 ),
 ( 1.570796326794896780, 3.141592653589793116 ),
 .UNSPECIFIED. ) 
 CURVE ( )  GEOMETRIC_REPRESENTATION_ITEM ( )  RATIONAL_B_SPLINE_CURVE ( ( 1.000000000000000000, 0.8047378541243650485, 0.8047378541243650485, 1.000000000000000000 ) ) 
 REPRESENTATION_ITEM ( '' )  );
#5219=ORIENTED_EDGE ( 'NONE', *, *, #4312, .F. ) ;
#5221=CARTESIAN_POINT ( 'NONE',  ( -55.00000000000000000, -10.00000000000000178, -17.50000000000000000 ) ) ;
#5229=DIRECTION ( 'NONE',  ( -0.4999999999999976685, -0.8660254037844399289, 0.000000000000000000 ) ) ;
#5238=CARTESIAN_POINT ( 'NONE',  ( -91.33974596215560382, -110.0591436588189396, 7.500000000000001776 ) ) ;
#5242=EDGE_CURVE ( 'NONE', #794, #14464, #15480, .T. ) ;
#5251=DIRECTION ( 'NONE',  ( -0.000000000000000000, -1.000000000000000000, -0.000000000000000000 ) ) ;
#5269=DIRECTION ( 'NONE',  ( 1.000000000000000000, 3.851859888774473808E-30, -1.387778780781445676E-15 ) ) ;
#5273=ORIENTED_EDGE ( 'NONE', *, *, #2, .F. ) ;
#5305=DIRECTION ( 'NONE',  ( -1.000000000000000000, 0.000000000000000000, 0.000000000000000000 ) ) ;
#5312=( BOUNDED_CURVE ( )  B_SPLINE_CURVE ( 3, ( #2060, #6691, #15496, #12885 ),
 .UNSPECIFIED., .F., .F. ) 
 B_SPLINE_CURVE_WITH_KNOTS ( ( 4, 4 ),
 ( 3.141592653589793116, 4.712388980384689674 ),
 .UNSPECIFIED. ) 
 CURVE ( )  GEOMETRIC_REPRESENTATION_ITEM ( )  RATIONAL_B_SPLINE_CURVE ( ( 1.000000000000000000, 0.8047378541243649375, 0.8047378541243649375, 1.000000000000000000 ) ) 
 REPRESENTATION_ITEM ( '' )  );
#5343=CIRCLE ( 'NONE', #14370, 10.00000000000000533 ) ;
#5374=DIRECTION ( 'NONE',  ( -0.000000000000000000, -1.000000000000000000, -0.000000000000000000 ) ) ;
#5376=VERTEX_POINT ( 'NONE', #630 ) ;
#5398=FACE_OUTER_BOUND ( 'NONE', #3723, .T. ) ;
#5399=DIRECTION ( 'NONE',  ( 0.000000000000000000, 0.000000000000000000, 1.000000000000000000 ) ) ;
#5435=EDGE_CURVE ( 'NONE', #1886, #15020, #2066, .T. ) ;
#5443=FACE_OUTER_BOUND ( 'NONE', #13159, .T. ) ;
#5447=EDGE_CURVE ( 'NONE', #6256, #14832, #9487, .T. ) ;
#5457=CARTESIAN_POINT ( 'NONE',  ( -90.00000000000000000, -95.00000000000000000, -7.500000000000000000 ) ) ;
#5466=DIRECTION ( 'NONE',  ( 0.4999999999999976685, 0.8660254037844399289, 0.000000000000000000 ) ) ;
#5474=VECTOR ( 'NONE', #5985, 1000.000000000000000 ) ;
#5493=DIRECTION ( 'NONE',  ( -6.938893903907228378E-16, -1.000000000000000000, 0.000000000000000000 ) ) ;
#5507=EDGE_CURVE ( 'NONE', #9005, #11530, #1743, .T. ) ;
#5513=CARTESIAN_POINT ( 'NONE',  ( -90.00000000000000000, -35.00000000000000711, -7.500000000000000000 ) ) ;
#5517=EDGE_LOOP ( 'NONE', ( #4779, #7091, #3818, #9863 ) ) ;
#5518=AXIS2_PLACEMENT_3D ( 'NONE', #6770, #15339, #15421 ) ;
#5523=ORIENTED_EDGE ( 'NONE', *, *, #15764, .F. ) ;
#5524=VECTOR ( 'NONE', #15556, 1000.000000000000000 ) ;
#5536=ADVANCED_FACE ( 'NONE', ( #14318 ), #9160, .T. ) ;
#5538=CARTESIAN_POINT ( 'NONE',  ( -39.99999999999999289, -13.00000000000000178, 8.300651832549021947E-13 ) ) ;
#5558=ORIENTED_EDGE ( 'NONE', *, *, #15347, .F. ) ;
#5560=COLOUR_RGB ( '', 0.09019608, 0.27058824, 0.51372549) ;
#5579=ORIENTED_EDGE ( 'NONE', *, *, #13823, .T. ) ;
#5594=VECTOR ( 'NONE', #8053, 1000.000000000000000 ) ;
#5608=ADVANCED_FACE ( 'NONE', ( #3399, #7217 ), #9698, .F. ) ;
#5616=VERTEX_POINT ( 'NONE', #3331 ) ;
#5646=LINE ( 'NONE', #15513, #5061 ) ;
#5680=EDGE_LOOP ( 'NONE', ( #10520, #6094, #2965, #7613 ) ) ;
#5683=EDGE_CURVE ( 'NONE', #6058, #8136, #7287, .T. ) ;
#5688=DIRECTION ( 'NONE',  ( -0.000000000000000000, -0.000000000000000000, -1.000000000000000000 ) ) ;
#5707=CARTESIAN_POINT ( 'NONE',  ( -36.99999999999999289, -13.00000000000000178, 2.000000000000830891 ) ) ;
#5727=CARTESIAN_POINT ( 'NONE',  ( -124.9999999999999716, -115.2072594216370049, 7.500000000000001776 ) ) ;
#5733=EDGE_LOOP ( 'NONE', ( #13560, #5558, #9741, #13054 ) ) ;
#5737=DIRECTION ( 'NONE',  ( -1.000000000000000000, -1.239088197126290324E-16, 0.000000000000000000 ) ) ;
#5739=EDGE_CURVE ( 'NONE', #12769, #6058, #4692, .T. ) ;
#5742=DIRECTION ( 'NONE',  ( 1.239088197126290324E-16, -1.000000000000000000, 0.000000000000000000 ) ) ;
#5770=ORIENTED_EDGE ( 'NONE', *, *, #4129, .F. ) ;
#5771=EDGE_LOOP ( 'NONE', ( #5852, #1815, #10324 ) ) ;
#5795=CARTESIAN_POINT ( 'NONE',  ( -124.9999999999999858, -115.2072594216369907, -7.500000000000000000 ) ) ;
#5807=ORIENTED_EDGE ( 'NONE', *, *, #13824, .F. ) ;
#5810=DIRECTION ( 'NONE',  ( 1.000000000000000000, -1.319090325525611458E-16, 0.000000000000000000 ) ) ;
#5811=VERTEX_POINT ( 'NONE', #3752 ) ;
#5814=CARTESIAN_POINT ( 'NONE',  ( -54.99999999999999289, -25.00000000000000000, -17.50000000000000000 ) ) ;
#5817=ORIENTED_EDGE ( 'NONE', *, *, #5507, .T. ) ;
#5821=CARTESIAN_POINT ( 'NONE',  ( -45.00000000000000000, -34.99999999999999289, 13.35786437626904899 ) ) ;
#5835=AXIS2_PLACEMENT_3D ( 'NONE', #14130, #11768, #13060 ) ;
#5838=AXIS2_PLACEMENT_3D ( 'NONE', #11406, #5269, #4054 ) ;
#5852=ORIENTED_EDGE ( 'NONE', *, *, #2589, .F. ) ;
#5871=ORIENTED_EDGE ( 'NONE', *, *, #15347, .T. ) ;
#5894=EDGE_LOOP ( 'NONE', ( #966, #373, #443 ) ) ;
#5901=FACE_OUTER_BOUND ( 'NONE', #8336, .T. ) ;
#5907=DIRECTION ( 'NONE',  ( 0.000000000000000000, 0.000000000000000000, 1.000000000000000000 ) ) ;
#5908=CARTESIAN_POINT ( 'NONE',  ( -115.0000000000000142, -10.00000000000000888, -7.500000000000000000 ) ) ;
#5909=CYLINDRICAL_SURFACE ( 'NONE', #7051, 9.999999999999994671 ) ;
#5918=ORIENTED_EDGE ( 'NONE', *, *, #1684, .F. ) ;
#5923=ADVANCED_FACE ( 'NONE', ( #7571 ), #2935, .T. ) ;
#5946=DIRECTION ( 'NONE',  ( 0.8660254037844405950, -0.4999999999999965028, -0.000000000000000000 ) ) ;
#5950=PLANE ( 'NONE',  #231 ) ;
#5962=FACE_OUTER_BOUND ( 'NONE', #14063, .T. ) ;
#5965=CARTESIAN_POINT ( 'NONE',  ( -124.9999999999999858, -115.2072594216369907, 7.500000000000001776 ) ) ;
#5972=VERTEX_POINT ( 'NONE', #9029 ) ;
#5979=ORIENTED_EDGE ( 'NONE', *, *, #1610, .T. ) ;
#5985=DIRECTION ( 'NONE',  ( 0.000000000000000000, 1.000000000000000000, -0.000000000000000000 ) ) ;
#6032=ORIENTED_EDGE ( 'NONE', *, *, #1261, .F. ) ;
#6040=LINE ( 'NONE', #12240, #15671 ) ;
#6058=VERTEX_POINT ( 'NONE', #5457 ) ;
#6067=VECTOR ( 'NONE', #8141, 1000.000000000000000 ) ;
#6091=DIRECTION ( 'NONE',  ( 0.000000000000000000, 0.000000000000000000, -1.000000000000000000 ) ) ;
#6094=ORIENTED_EDGE ( 'NONE', *, *, #6240, .T. ) ;
#6106=FILL_AREA_STYLE_COLOUR ( '', #11575 ) ;
#6139=CARTESIAN_POINT ( 'NONE',  ( -99.99999999999998579, -100.7735026918962831, -17.50000000000000000 ) ) ;
#6150=CARTESIAN_POINT ( 'NONE',  ( -158.0560796608385488, -84.57531754730580076, -17.50000000000000000 ) ) ;
#6156=CARTESIAN_POINT ( 'NONE',  ( -124.9999999999999716, -10.00000000000001066, 7.500000000000001776 ) ) ;
#6165=VERTEX_POINT ( 'NONE', #15320 ) ;
#6180=ORIENTED_EDGE ( 'NONE', *, *, #979, .T. ) ;
#6182=ORIENTED_EDGE ( 'NONE', *, *, #14524, .F. ) ;
#6211=CARTESIAN_POINT ( 'NONE',  ( -113.6871902368263250, -110.1917077999037957, 17.50000000000000000 ) ) ;
#6230=LINE ( 'NONE', #13467, #6797 ) ;
#6232=CARTESIAN_POINT ( 'NONE',  ( -99.99999999999998579, -35.00000000000000711, -7.500000000000000000 ) ) ;
#6240=EDGE_CURVE ( 'NONE', #7722, #11193, #11017, .T. ) ;
#6256=VERTEX_POINT ( 'NONE', #4637 ) ;
#6257=CYLINDRICAL_SURFACE ( 'NONE', #13138, 9.999999999999994671 ) ;
#6266=DIRECTION ( 'NONE',  ( -1.000000000000000000, -1.982541115402064863E-16, 0.000000000000000000 ) ) ;
#6268=CARTESIAN_POINT ( 'NONE',  ( -44.99999999999999289, -35.00000000000000000, -7.500000000000000000 ) ) ;
#6280=ORIENTED_EDGE ( 'NONE', *, *, #12050, .F. ) ;
#6302=DIRECTION ( 'NONE',  ( 0.000000000000000000, -1.387778780781445676E-15, -1.000000000000000000 ) ) ;
#6306=EDGE_CURVE ( 'NONE', #6165, #9005, #3490, .T. ) ;
#6347=AXIS2_PLACEMENT_3D ( 'NONE', #13310, #1046, #15844 ) ;
#6384=AXIS2_PLACEMENT_3D ( 'NONE', #2549, #5305, #13942 ) ;
#6388=DIRECTION ( 'NONE',  ( 1.000000000000000000, 0.000000000000000000, 0.000000000000000000 ) ) ;
#6392=DIRECTION ( 'NONE',  ( 1.000000000000000000, -6.938893903907232322E-16, 0.000000000000000000 ) ) ;
#6439=DIRECTION ( 'NONE',  ( 1.000000000000000000, 1.734723475976806848E-16, 0.000000000000000000 ) ) ;
#6447=ORIENTED_EDGE ( 'NONE', *, *, #586, .F. ) ;
#6456=LINE ( 'NONE', #2555, #11811 ) ;
#6484=EDGE_LOOP ( 'NONE', ( #2762, #10627, #3756 ) ) ;
#6495=ORIENTED_EDGE ( 'NONE', *, *, #11960, .T. ) ;
#6513=CARTESIAN_POINT ( 'NONE',  ( -55.00000000000000000, -9.999999999999996447, 7.500000000000001776 ) ) ;
#6534=LINE ( 'NONE', #14208, #14606 ) ;
#6538=DIRECTION ( 'NONE',  ( -0.000000000000000000, -1.000000000000000000, -0.000000000000000000 ) ) ;
#6556=ORIENTED_EDGE ( 'NONE', *, *, #12301, .T. ) ;
#6577=EDGE_CURVE ( 'NONE', #4817, #7310, #4926, .T. ) ;
#6603=FACE_OUTER_BOUND ( 'NONE', #5164, .T. ) ;
#6615=ORIENTED_EDGE ( 'NONE', *, *, #2752, .T. ) ;
#6622=ADVANCED_FACE ( 'NONE', ( #15848 ), #2256, .T. ) ;
#6623=ORIENTED_EDGE ( 'NONE', *, *, #3033, .F. ) ;
#6671=EDGE_CURVE ( 'NONE', #9599, #6256, #7773, .T. ) ;
#6673=VECTOR ( 'NONE', #1734, 1000.000000000000000 ) ;
#6691=CARTESIAN_POINT ( 'NONE',  ( -116.3391301858327012, -120.2076149402627010, -13.35786437626904721 ) ) ;
#6694=CARTESIAN_POINT ( 'NONE',  ( -81.33974596215558961, -99.99999999999995737, 17.50000000000000000 ) ) ;
#6696=CYLINDRICAL_SURFACE ( 'NONE', #2133, 10.00000000000000000 ) ;
#6741=DIRECTION ( 'NONE',  ( -0.000000000000000000, -0.000000000000000000, -1.000000000000000000 ) ) ;
#6745=LINE ( 'NONE', #13918, #10582 ) ;
#6752=CARTESIAN_POINT ( 'NONE',  ( -81.33974596215560382, -110.0591436588189538, 17.50000000000000000 ) ) ;
#6759=VERTEX_POINT ( 'NONE', #13428 ) ;
#6762=ORIENTED_EDGE ( 'NONE', *, *, #3515, .T. ) ;
#6770=CARTESIAN_POINT ( 'NONE',  ( -36.99999999999999289, -13.00000000000000178, -1.999999999999170885 ) ) ;
#6774=EDGE_LOOP ( 'NONE', ( #14083, #2920, #5199 ) ) ;
#6793=CARTESIAN_POINT ( 'NONE',  ( -34.99999999999999289, -13.00000000000000178, 2.000000000000830447 ) ) ;
#6794=ORIENTED_EDGE ( 'NONE', *, *, #8418, .F. ) ;
#6797=VECTOR ( 'NONE', #4766, 1000.000000000000000 ) ;
#6817=EDGE_CURVE ( 'NONE', #1886, #658, #15464, .T. ) ;
#6820=CARTESIAN_POINT ( 'NONE',  ( -99.99999999999998579, -100.7735026918962831, -17.50000000000000000 ) ) ;
#6841=CARTESIAN_POINT ( 'NONE',  ( -36.99999999999999289, -11.00000000000000178, 2.000000000000830891 ) ) ;
#6888=AXIS2_PLACEMENT_3D ( 'NONE', #9055, #6538, #13880 ) ;
#6911=DIRECTION ( 'NONE',  ( 0.000000000000000000, 0.000000000000000000, -1.000000000000000000 ) ) ;
#6946=AXIS2_PLACEMENT_3D ( 'NONE', #4949, #1306, #11097 ) ;
#6973=ADVANCED_BREP_SHAPE_REPRESENTATION ( '', ( #3386, #3223 ), #1155 ) ;
#6983=CARTESIAN_POINT ( 'NONE',  ( -115.0000000000000142, -10.00000000000000888, 7.500000000000001776 ) ) ;
#6992=LINE ( 'NONE', #10553, #5524 ) ;
#7018=EDGE_LOOP ( 'NONE', ( #8770, #6447, #8173, #5770 ) ) ;
#7020=EDGE_LOOP ( 'NONE', ( #14515, #10540, #10302, #4217, #5979, #2639, #4756, #7595, #8104 ) ) ;
#7045=DIRECTION ( 'NONE',  ( -1.541976423090495140E-16, 1.000000000000000000, 0.000000000000000000 ) ) ;
#7048=DIRECTION ( 'NONE',  ( 1.000000000000000000, 1.541976423090495140E-16, -0.000000000000000000 ) ) ;
#7049=LINE ( 'NONE', #14241, #8500 ) ;
#7051=AXIS2_PLACEMENT_3D ( 'NONE', #10835, #11710, #4529 ) ;
#7059=EDGE_CURVE ( 'NONE', #658, #7410, #8756, .T. ) ;
#7069=CIRCLE ( 'NONE', #5518, 2.000000000000000888 ) ;
#7073=DIRECTION ( 'NONE',  ( -1.319090325525611458E-16, -1.000000000000000000, 0.000000000000000000 ) ) ;
#7076=DIRECTION ( 'NONE',  ( 1.319090325525611458E-16, 1.000000000000000000, -0.000000000000000000 ) ) ;
#7078=AXIS2_PLACEMENT_3D ( 'NONE', #7652, #7566, #15153 ) ;
#7081=DIRECTION ( 'NONE',  ( 0.000000000000000000, 0.000000000000000000, 1.000000000000000000 ) ) ;
#7089=AXIS2_PLACEMENT_3D ( 'NONE', #7776, #5493, #6392 ) ;
#7091=ORIENTED_EDGE ( 'NONE', *, *, #3407, .F. ) ;
#7123=CIRCLE ( 'NONE', #155, 2.000000000000000888 ) ;
#7138=ORIENTED_EDGE ( 'NONE', *, *, #586, .T. ) ;
#7147=CIRCLE ( 'NONE', #14110, 10.00000000000000711 ) ;
#7156=FACE_OUTER_BOUND ( 'NONE', #15897, .T. ) ;
#7163=CARTESIAN_POINT ( 'NONE',  ( -86.33974596215563224, -97.11324865405184426, 7.500000000000001776 ) ) ;
#7180=VERTEX_POINT ( 'NONE', #7298 ) ;
#7198=CARTESIAN_POINT ( 'NONE',  ( -114.9999999999999858, -109.4337567297407219, 17.50000000000000000 ) ) ;
#7206=CYLINDRICAL_SURFACE ( 'NONE', #6347, 10.00000000000000711 ) ;
#7208=CARTESIAN_POINT ( 'NONE',  ( -44.99999999999999289, -11.00000000000000178, -3.999999999999170885 ) ) ;
#7210=LINE ( 'NONE', #2485, #15825 ) ;
#7217=FACE_BOUND ( 'NONE', #12920, .T. ) ;
#7235=DIRECTION ( 'NONE',  ( -6.938893903907228378E-16, -1.000000000000000000, -0.000000000000000000 ) ) ;
#7273=CARTESIAN_POINT ( 'NONE',  ( -99.99999999999998579, -25.00000000000000711, -17.50000000000000000 ) ) ;
#7279=LINE ( 'NONE', #12027, #1255 ) ;
#7287=LINE ( 'NONE', #15702, #11039 ) ;
#7298=CARTESIAN_POINT ( 'NONE',  ( -91.33974596215558961, -105.7735026918962404, -17.50000000000000000 ) ) ;
#7303=DIRECTION ( 'NONE',  ( 0.000000000000000000, 0.000000000000000000, 1.000000000000000000 ) ) ;
#7310=VERTEX_POINT ( 'NONE', #2084 ) ;
#7319=( NAMED_UNIT ( * ) PLANE_ANGLE_UNIT ( ) SI_UNIT ( $, .RADIAN. ) );
#7336=DIRECTION ( 'NONE',  ( 0.000000000000000000, 0.000000000000000000, 1.000000000000000000 ) ) ;
#7353=EDGE_LOOP ( 'NONE', ( #7138, #7895, #1148, #564 ) ) ;
#7360=DIRECTION ( 'NONE',  ( 0.000000000000000000, 1.000000000000000000, -0.000000000000000000 ) ) ;
#7368=ORIENTED_EDGE ( 'NONE', *, *, #5447, .F. ) ;
#7393=DIRECTION ( 'NONE',  ( -0.000000000000000000, -0.000000000000000000, -1.000000000000000000 ) ) ;
#7404=AXIS2_PLACEMENT_3D ( 'NONE', #8478, #14689, #12087 ) ;
#7410=VERTEX_POINT ( 'NONE', #238 ) ;
#7411=AXIS2_PLACEMENT_3D ( 'NONE', #7208, #5907, #1203 ) ;
#7420=CARTESIAN_POINT ( 'NONE',  ( -36.99999999999999289, -13.00000000000000178, -3.999999999999170885 ) ) ;
#7423=ADVANCED_FACE ( 'NONE', ( #1515 ), #8957, .F. ) ;
#7446=EDGE_CURVE ( 'NONE', #15896, #15795, #1905, .T. ) ;
#7448=DIRECTION ( 'NONE',  ( 1.000000000000000000, -1.734723475976808080E-16, 0.000000000000000000 ) ) ;
#7449=APPLICATION_CONTEXT ( 'automotive_design' ) ;
#7455=ORIENTED_EDGE ( 'NONE', *, *, #1060, .F. ) ;
#7458=LINE ( 'NONE', #3477, #160 ) ;
#7459=AXIS2_PLACEMENT_3D ( 'NONE', #11288, #2800, #11204 ) ;
#7479=CYLINDRICAL_SURFACE ( 'NONE', #8659, 9.999999999999980460 ) ;
#7485=LINE ( 'NONE', #6268, #1242 ) ;
#7488=ORIENTED_EDGE ( 'NONE', *, *, #12350, .F. ) ;
#7501=EDGE_CURVE ( 'NONE', #4500, #13155, #15173, .T. ) ;
#7511=ORIENTED_EDGE ( 'NONE', *, *, #9325, .F. ) ;
#7519=EDGE_CURVE ( 'NONE', #757, #794, #2712, .T. ) ;
#7521=FACE_OUTER_BOUND ( 'NONE', #15343, .T. ) ;
#7566=DIRECTION ( 'NONE',  ( 0.000000000000000000, 1.000000000000000000, 0.000000000000000000 ) ) ;
#7571=FACE_OUTER_BOUND ( 'NONE', #393, .T. ) ;
#7577=ORIENTED_EDGE ( 'NONE', *, *, #15764, .T. ) ;
#7585=CARTESIAN_POINT ( 'NONE',  ( -54.99999999999999289, -25.00000000000000000, -17.50000000000000000 ) ) ;
#7588=ADVANCED_FACE ( 'NONE', ( #317 ), #15258, .F. ) ;
#7592=ORIENTED_EDGE ( 'NONE', *, *, #3648, .F. ) ;
#7593=DIRECTION ( 'NONE',  ( 0.000000000000000000, 0.000000000000000000, -1.000000000000000000 ) ) ;
#7595=ORIENTED_EDGE ( 'NONE', *, *, #10842, .T. ) ;
#7613=ORIENTED_EDGE ( 'NONE', *, *, #13802, .T. ) ;
#7640=ORIENTED_EDGE ( 'NONE', *, *, #13097, .F. ) ;
#7646=CARTESIAN_POINT ( 'NONE',  ( -45.00000000000000000, 0.000000000000000000, -7.500000000000000000 ) ) ;
#7652=CARTESIAN_POINT ( 'NONE',  ( -91.33974596215560382, -110.0591436588189396, -7.500000000000001776 ) ) ;
#7654=DIRECTION ( 'NONE',  ( -1.387778780781446464E-15, -1.000000000000000000, 1.387778780781445478E-15 ) ) ;
#7664=AXIS2_PLACEMENT_3D ( 'NONE', #5238, #486, #6302 ) ;
#7683=ORIENTED_EDGE ( 'NONE', *, *, #10414, .T. ) ;
#7687=EDGE_CURVE ( 'NONE', #794, #11044, #8297, .T. ) ;
#7689=DIRECTION ( 'NONE',  ( -1.000000000000000000, -1.541976423090495140E-16, 0.000000000000000000 ) ) ;
#7691=FACE_OUTER_BOUND ( 'NONE', #4883, .T. ) ;
#7695=DIRECTION ( 'NONE',  ( 0.000000000000000000, 0.000000000000000000, -1.000000000000000000 ) ) ;
#7722=VERTEX_POINT ( 'NONE', #15418 ) ;
#7773=LINE ( 'NONE', #15105, #10799 ) ;
#7776=CARTESIAN_POINT ( 'NONE',  ( -91.33974596215551855, -10.00000000000002487, 7.500000000000001776 ) ) ;
#7797=SURFACE_STYLE_FILL_AREA ( #12616 ) ;
#7841=CYLINDRICAL_SURFACE ( 'NONE', #6888, 2.500000000000909495 ) ;
#7870=( NAMED_UNIT ( * ) PLANE_ANGLE_UNIT ( ) SI_UNIT ( $, .RADIAN. ) );
#7872=CARTESIAN_POINT ( 'NONE',  ( -115.0000000000000000, -10.00000000000000888, -7.500000000000000000 ) ) ;
#7894=DIRECTION ( 'NONE',  ( -0.000000000000000000, -0.000000000000000000, -1.000000000000000000 ) ) ;
#7895=ORIENTED_EDGE ( 'NONE', *, *, #4216, .T. ) ;
#7911=VECTOR ( 'NONE', #15402, 1000.000000000000000 ) ;
#7928=AXIS2_PLACEMENT_3D ( 'NONE', #12401, #11435, #310 ) ;
#7932=DIRECTION ( 'NONE',  ( -1.000000000000000000, 0.000000000000000000, 0.000000000000000000 ) ) ;
#7935=CARTESIAN_POINT ( 'NONE',  ( -45.00000000000000000, 0.000000000000000000, 7.500000000000001776 ) ) ;
#7970=EDGE_LOOP ( 'NONE', ( #8991, #3913, #4714, #1702 ) ) ;
#7973=VECTOR ( 'NONE', #7073, 1000.000000000000000 ) ;
#7976=ORIENTED_EDGE ( 'NONE', *, *, #8376, .T. ) ;
#7978=ORIENTED_EDGE ( 'NONE', *, *, #10842, .F. ) ;
#7980=CYLINDRICAL_SURFACE ( 'NONE', #9383, 2.000000000000000888 ) ;
#8026=VERTEX_POINT ( 'NONE', #11266 ) ;
#8031=CARTESIAN_POINT ( 'NONE',  ( -90.00000000000000000, -95.00000000000000000, 7.500000000000001776 ) ) ;
#8038=ADVANCED_FACE ( 'NONE', ( #47 ), #3746, .T. ) ;
#8043=ORIENTED_EDGE ( 'NONE', *, *, #7519, .F. ) ;
#8050=DIRECTION ( 'NONE',  ( 0.000000000000000000, -0.000000000000000000, -1.000000000000000000 ) ) ;
#8051=EDGE_LOOP ( 'NONE', ( #12733, #6794, #8678, #7455 ) ) ;
#8053=DIRECTION ( 'NONE',  ( -0.8660254037844405950, 0.4999999999999965028, 0.000000000000000000 ) ) ;
#8058=ORIENTED_EDGE ( 'NONE', *, *, #3562, .F. ) ;
#8060=CARTESIAN_POINT ( 'NONE',  ( -36.99999999999999289, -11.00000000000000178, 2.000000000000830891 ) ) ;
#8079=ORIENTED_EDGE ( 'NONE', *, *, #3515, .F. ) ;
#8104=ORIENTED_EDGE ( 'NONE', *, *, #6577, .T. ) ;
#8108=EDGE_CURVE ( 'NONE', #5616, #1597, #7049, .T. ) ;
#8117=DIRECTION ( 'NONE',  ( 0.000000000000000000, 1.000000000000000000, 0.000000000000000000 ) ) ;
#8128=FACE_OUTER_BOUND ( 'NONE', #14948, .T. ) ;
#8132=LINE ( 'NONE', #14188, #5594 ) ;
#8135=DIRECTION ( 'NONE',  ( -0.9999824063907751803, -0.005931855436079011210, 0.000000000000000000 ) ) ;
#8136=VERTEX_POINT ( 'NONE', #5513 ) ;
#8137=VECTOR ( 'NONE', #2567, 1000.000000000000000 ) ;
#8141=DIRECTION ( 'NONE',  ( 1.319090325525611458E-16, 1.000000000000000000, -0.000000000000000000 ) ) ;
#8169=FACE_OUTER_BOUND ( 'NONE', #770, .T. ) ;
#8173=ORIENTED_EDGE ( 'NONE', *, *, #1181, .F. ) ;
#8192=DIRECTION ( 'NONE',  ( 6.938893903907228378E-16, 1.000000000000000000, -0.000000000000000000 ) ) ;
#8196=( NAMED_UNIT ( * ) SI_UNIT ( $, .STERADIAN. ) SOLID_ANGLE_UNIT ( ) );
#8256=AXIS2_PLACEMENT_3D ( 'NONE', #2099, #7045, #7689 ) ;
#8273=AXIS2_PLACEMENT_3D ( 'NONE', #6983, #8117, #13012 ) ;
#8274=PLANE ( 'NONE',  #8256 ) ;
#8275=CARTESIAN_POINT ( 'NONE',  ( -45.00000000000000000, 0.000000000000000000, -7.500000000000000000 ) ) ;
#8283=ORIENTED_EDGE ( 'NONE', *, *, #10428, .F. ) ;
#8297=LINE ( 'NONE', #15562, #11510 ) ;
#8333=ORIENTED_EDGE ( 'NONE', *, *, #4109, .T. ) ;
#8335=ORIENTED_EDGE ( 'NONE', *, *, #2948, .T. ) ;
#8336=EDGE_LOOP ( 'NONE', ( #7683, #14304, #8863, #6495 ) ) ;
#8345=CARTESIAN_POINT ( 'NONE',  ( -44.99999999999998579, -25.00000000000000000, 17.50000000000000000 ) ) ;
#8350=VECTOR ( 'NONE', #2370, 1000.000000000000000 ) ;
#8358=EDGE_CURVE ( 'NONE', #5811, #8026, #10780, .T. ) ;
#8376=EDGE_CURVE ( 'NONE', #11044, #12769, #15110, .T. ) ;
#8400=SPHERICAL_SURFACE ( 'NONE', #7404, 10.00000000000000000 ) ;
#8418=EDGE_CURVE ( 'NONE', #6759, #2789, #11464, .T. ) ;
#8423=CARTESIAN_POINT ( 'NONE',  ( -44.99999999999999289, -13.00000000000000178, 4.000000000000831335 ) ) ;
#8431=CARTESIAN_POINT ( 'NONE',  ( -91.33974596215558961, -99.99999999999994316, -7.500000000000000000 ) ) ;
#8468=VECTOR ( 'NONE', #13321, 1000.000000000000000 ) ;
#8474=VECTOR ( 'NONE', #5251, 1000.000000000000000 ) ;
#8475=DIRECTION ( 'NONE',  ( 0.000000000000000000, 0.000000000000000000, 1.000000000000000000 ) ) ;
#8478=CARTESIAN_POINT ( 'NONE',  ( -91.33974596215558961, -105.7735026918962404, -7.500000000000001776 ) ) ;
#8491=FACE_OUTER_BOUND ( 'NONE', #5680, .T. ) ;
#8500=VECTOR ( 'NONE', #9469, 1000.000000000000000 ) ;
#8505=DIRECTION ( 'NONE',  ( 0.9999824063907751803, 0.005931855436079011210, -0.000000000000000000 ) ) ;
#8518=CARTESIAN_POINT ( 'NONE',  ( -90.00000000000000000, -35.00000000000000000, 13.35786437626905077 ) ) ;
#8532=ORIENTED_EDGE ( 'NONE', *, *, #8862, .F. ) ;
#8557=DIRECTION ( 'NONE',  ( 0.4999999999999960032, 0.8660254037844409281, 0.000000000000000000 ) ) ;
#8601=DIRECTION ( 'NONE',  ( -1.000000000000000000, 0.000000000000000000, 0.000000000000000000 ) ) ;
#8606=EDGE_CURVE ( 'NONE', #15795, #3371, #807, .T. ) ;
#8613=AXIS2_PLACEMENT_3D ( 'NONE', #10002, #9756, #2466 ) ;
#8642=EDGE_LOOP ( 'NONE', ( #8335, #1736, #7511, #4624 ) ) ;
#8656=CYLINDRICAL_SURFACE ( 'NONE', #1395, 9.999999999999994671 ) ;
#8659=AXIS2_PLACEMENT_3D ( 'NONE', #9016, #5128, #11262 ) ;
#8675=CARTESIAN_POINT ( 'NONE',  ( -115.0000000000000142, -10.00000000000000888, -17.50000000000000000 ) ) ;
#8678=ORIENTED_EDGE ( 'NONE', *, *, #11551, .F. ) ;
#8683=FACE_OUTER_BOUND ( 'NONE', #7018, .T. ) ;
#8703=FACE_OUTER_BOUND ( 'NONE', #5517, .T. ) ;
#8714=DIRECTION ( 'NONE',  ( -0.000000000000000000, -1.000000000000000000, 0.000000000000000000 ) ) ;
#8737=CARTESIAN_POINT ( 'NONE',  ( -91.33974596215558961, -105.7735026918962262, 7.500000000000001776 ) ) ;
#8756=CIRCLE ( 'NONE', #13114, 9.999999999999980460 ) ;
#8770=ORIENTED_EDGE ( 'NONE', *, *, #8358, .F. ) ;
#8809=EDGE_LOOP ( 'NONE', ( #1117, #4402, #11901, #3438 ) ) ;
#8820=LINE ( 'NONE', #15932, #5474 ) ;
#8838=DIRECTION ( 'NONE',  ( -0.000000000000000000, -1.000000000000000000, -0.000000000000000000 ) ) ;
#8843=DIRECTION ( 'NONE',  ( 1.734723475976808080E-16, -1.000000000000000000, -2.407412430484045692E-31 ) ) ;
#8844=DIRECTION ( 'NONE',  ( -0.000000000000000000, -1.000000000000000000, -0.000000000000000000 ) ) ;
#8862=EDGE_CURVE ( 'NONE', #7310, #6759, #6456, .T. ) ;
#8863=ORIENTED_EDGE ( 'NONE', *, *, #2752, .F. ) ;
#8870=VECTOR ( 'NONE', #3690, 1000.000000000000000 ) ;
#8876=CARTESIAN_POINT ( 'NONE',  ( -39.99999999999999289, -11.00000000000000178, 2.500000000001739497 ) ) ;
#8879=EDGE_LOOP ( 'NONE', ( #2332, #9585, #9326, #696 ) ) ;
#8889=VERTEX_POINT ( 'NONE', #8876 ) ;
#8910=ORIENTED_EDGE ( 'NONE', *, *, #2948, .F. ) ;
#8927=CARTESIAN_POINT ( 'NONE',  ( -36.99999999999999289, -11.00000000000000178, -3.999999999999170885 ) ) ;
#8938=DIRECTION ( 'NONE',  ( 1.000000000000000000, 1.541976423090495140E-16, -0.000000000000000000 ) ) ;
#8952=CIRCLE ( 'NONE', #15666, 10.00000000000000711 ) ;
#8957=PLANE ( 'NONE',  #7459 ) ;
#8969=FACE_OUTER_BOUND ( 'NONE', #8879, .T. ) ;
#8977=DIRECTION ( 'NONE',  ( -0.000000000000000000, -1.000000000000000000, -0.000000000000000000 ) ) ;
#8991=ORIENTED_EDGE ( 'NONE', *, *, #10294, .T. ) ;
#9005=VERTEX_POINT ( 'NONE', #15577 ) ;
#9016=CARTESIAN_POINT ( 'NONE',  ( -115.0000000000000142, -10.00000000000000888, 17.50000000000000000 ) ) ;
#9029=CARTESIAN_POINT ( 'NONE',  ( -44.99999999999999289, -11.00000000000000178, 4.000000000000831335 ) ) ;
#9035=VECTOR ( 'NONE', #7894, 1000.000000000000000 ) ;
#9042=DIRECTION ( 'NONE',  ( -1.000000000000000000, 6.938893903907228378E-16, 0.000000000000000000 ) ) ;
#9054=ADVANCED_FACE ( 'NONE', ( #5398 ), #4344, .T. ) ;
#9055=CARTESIAN_POINT ( 'NONE',  ( -39.99999999999999289, -11.00000000000000178, 8.300651832549021947E-13 ) ) ;
#9058=( BOUNDED_CURVE ( )  B_SPLINE_CURVE ( 3, ( #5795, #10731, #4742, #2315 ),
 .UNSPECIFIED., .F., .F. ) 
 B_SPLINE_CURVE_WITH_KNOTS ( ( 4, 4 ),
 ( 3.141592653589793116, 4.712388980384689674 ),
 .UNSPECIFIED. ) 
 CURVE ( )  GEOMETRIC_REPRESENTATION_ITEM ( )  RATIONAL_B_SPLINE_CURVE ( ( 1.000000000000000000, 0.8047378541243649375, 0.8047378541243649375, 1.000000000000000000 ) ) 
 REPRESENTATION_ITEM ( '' )  );
#9089=ADVANCED_FACE ( 'NONE', ( #3201 ), #5950, .F. ) ;
#9119=FACE_OUTER_BOUND ( 'NONE', #619, .T. ) ;
#9151=( BOUNDED_CURVE ( )  B_SPLINE_CURVE ( 3, ( #15785, #8518, #2496, #4780 ),
 .UNSPECIFIED., .F., .F. ) 
 B_SPLINE_CURVE_WITH_KNOTS ( ( 4, 4 ),
 ( 3.141592653589793116, 4.712388980384689674 ),
 .UNSPECIFIED. ) 
 CURVE ( )  GEOMETRIC_REPRESENTATION_ITEM ( )  RATIONAL_B_SPLINE_CURVE ( ( 1.000000000000000000, 0.8047378541243649375, 0.8047378541243649375, 1.000000000000000000 ) ) 
 REPRESENTATION_ITEM ( '' )  );
#9159=AXIS2_PLACEMENT_3D ( 'NONE', #10661, #3305, #11931 ) ;
#9160=CYLINDRICAL_SURFACE ( 'NONE', #11556, 9.999999999999998224 ) ;
#9167=CIRCLE ( 'NONE', #4773, 2.000000000000000888 ) ;
#9181=DIRECTION ( 'NONE',  ( -0.000000000000000000, -0.000000000000000000, 1.000000000000000000 ) ) ;
#9191=AXIS2_PLACEMENT_3D ( 'NONE', #10525, #13085, #11872 ) ;
#9200=CARTESIAN_POINT ( 'NONE',  ( -99.99999999999998579, -10.00000000000000888, 7.500000000000001776 ) ) ;
#9261=CARTESIAN_POINT ( 'NONE',  ( -44.99999999999999289, -11.00000000000000178, 4.000000000000831335 ) ) ;
#9284=CIRCLE ( 'NONE', #11330, 2.500000000000909495 ) ;
#9293=ORIENTED_EDGE ( 'NONE', *, *, #11352, .F. ) ;
#9295=AXIS2_PLACEMENT_3D ( 'NONE', #3659, #112, #5034 ) ;
#9296=CARTESIAN_POINT ( 'NONE',  ( -55.00000000000000000, -10.00000000000000178, 17.50000000000000000 ) ) ;
#9301=DIRECTION ( 'NONE',  ( -0.000000000000000000, -0.000000000000000000, -1.000000000000000000 ) ) ;
#9312=ADVANCED_FACE ( 'NONE', ( #8128 ), #1884, .T. ) ;
#9315=DIRECTION ( 'NONE',  ( 1.000000000000000000, 1.239088197126290324E-16, 0.000000000000000000 ) ) ;
#9325=EDGE_CURVE ( 'NONE', #14420, #4500, #15397, .T. ) ;
#9326=ORIENTED_EDGE ( 'NONE', *, *, #4746, .F. ) ;
#9332=LINE ( 'NONE', #14096, #10074 ) ;
#9358=UNCERTAINTY_MEASURE_WITH_UNIT (LENGTH_MEASURE( 1.000000000000000082E-05 ), #13509, 'distance_accuracy_value', 'NONE');
#9365=VECTOR ( 'NONE', #9611, 1000.000000000000000 ) ;
#9383=AXIS2_PLACEMENT_3D ( 'NONE', #8060, #1893, #2058 ) ;
#9398=EDGE_LOOP ( 'NONE', ( #12391, #11000, #5219, #7976 ) ) ;
#9424=CARTESIAN_POINT ( 'NONE',  ( -115.0000000000000142, -10.00000000000000888, 17.50000000000000000 ) ) ;
#9459=CARTESIAN_POINT ( 'NONE',  ( -115.0000000000000142, -10.00000000000000888, 17.50000000000000000 ) ) ;
#9469=DIRECTION ( 'NONE',  ( 6.938893903907228378E-16, 1.000000000000000000, -0.000000000000000000 ) ) ;
#9480=EDGE_CURVE ( 'NONE', #2808, #14971, #14981, .T. ) ;
#9482=DIRECTION ( 'NONE',  ( -1.000000000000000000, 0.000000000000000000, 0.000000000000000000 ) ) ;
#9487=CIRCLE ( 'NONE', #466, 2.000000000000000888 ) ;
#9491=LINE ( 'NONE', #617, #13840 ) ;
#9499=ADVANCED_FACE ( 'NONE', ( #1226 ), #3817, .T. ) ;
#9500=CARTESIAN_POINT ( 'NONE',  ( -90.00000000000000000, -35.00000000000000711, -7.500000000000000000 ) ) ;
#9503=CARTESIAN_POINT ( 'NONE',  ( -34.99999999999999289, -13.00000000000000178, -1.999999999999170441 ) ) ;
#9504=CARTESIAN_POINT ( 'NONE',  ( -39.99999999999999289, -13.00000000000000178, 8.300651832549021947E-13 ) ) ;
#9506=AXIS2_PLACEMENT_3D ( 'NONE', #5908, #13642, #12028 ) ;
#9518=PRODUCT ( 'Synchronized Concentric Jaws', 'Synchronized Concentric Jaws', '', ( #2592 ) ) ;
#9536=ORIENTED_EDGE ( 'NONE', *, *, #6817, .T. ) ;
#9543=AXIS2_PLACEMENT_3D ( 'NONE', #2055, #8135, #12954 ) ;
#9567=ORIENTED_EDGE ( 'NONE', *, *, #10365, .F. ) ;
#9573=CARTESIAN_POINT ( 'NONE',  ( -115.0000000000000142, -10.00000000000000888, 17.50000000000000000 ) ) ;
#9585=ORIENTED_EDGE ( 'NONE', *, *, #3562, .T. ) ;
#9599=VERTEX_POINT ( 'NONE', #8423 ) ;
#9611=DIRECTION ( 'NONE',  ( -1.000000000000000000, -1.239088197126290324E-16, 0.000000000000000000 ) ) ;
#9617=DIRECTION ( 'NONE',  ( 0.000000000000000000, -1.000000000000000000, 0.000000000000000000 ) ) ;
#9632=FACE_OUTER_BOUND ( 'NONE', #9398, .T. ) ;
#9638=CARTESIAN_POINT ( 'NONE',  ( -91.33974596215560382, -110.0591436588189396, -7.500000000000000000 ) ) ;
#9650=CARTESIAN_POINT ( 'NONE',  ( -124.9999999999999858, -115.2072594216369907, 7.500000000000001776 ) ) ;
#9673=( GEOMETRIC_REPRESENTATION_CONTEXT ( 3 ) GLOBAL_UNCERTAINTY_ASSIGNED_CONTEXT ( ( #4961 ) ) GLOBAL_UNIT_ASSIGNED_CONTEXT ( ( #4539, #4305, #8196 ) ) REPRESENTATION_CONTEXT ( 'NONE', 'WORKASPACE' ) );
#9676=VECTOR ( 'NONE', #11733, 1000.000000000000000 ) ;
#9686=EDGE_CURVE ( 'NONE', #15795, #11117, #7279, .T. ) ;
#9698=PLANE ( 'NONE',  #15437 ) ;
#9700=ORIENTED_EDGE ( 'NONE', *, *, #15417, .F. ) ;
#9707=ADVANCED_FACE ( 'NONE', ( #4610 ), #4684, .F. ) ;
#9739=DIRECTION ( 'NONE',  ( 0.000000000000000000, 1.000000000000000000, 0.000000000000000000 ) ) ;
#9741=ORIENTED_EDGE ( 'NONE', *, *, #13823, .F. ) ;
#9756=DIRECTION ( 'NONE',  ( -0.000000000000000000, -0.000000000000000000, 1.000000000000000000 ) ) ;
#9762=ORIENTED_EDGE ( 'NONE', *, *, #2042, .T. ) ;
#9765=ORIENTED_EDGE ( 'NONE', *, *, #10774, .F. ) ;
#9766=ADVANCED_FACE ( 'NONE', ( #14784 ), #8274, .F. ) ;
#9781=CYLINDRICAL_SURFACE ( 'NONE', #645, 10.00000000000000000 ) ;
#9797=CARTESIAN_POINT ( 'NONE',  ( -90.00000000000000000, -34.99999999999999289, -13.35786437626904899 ) ) ;
#9804=CARTESIAN_POINT ( 'NONE',  ( -39.99999999999999289, -11.00000000000000178, -2.500000000000079492 ) ) ;
#9812=LINE ( 'NONE', #9503, #13791 ) ;
#9832=CARTESIAN_POINT ( 'NONE',  ( -120.8578643762690490, -112.8157963042559544, 17.49999999999999289 ) ) ;
#9839=( BOUNDED_CURVE ( )  B_SPLINE_CURVE ( 3, ( #13239, #5821, #11873, #820 ),
 .UNSPECIFIED., .F., .T. ) 
 B_SPLINE_CURVE_WITH_KNOTS ( ( 4, 4 ),
 ( 0.000000000000000000, 1.570796326794896336 ),
 .UNSPECIFIED. ) 
 CURVE ( )  GEOMETRIC_REPRESENTATION_ITEM ( )  RATIONAL_B_SPLINE_CURVE ( ( 1.000000000000000000, 0.8047378541243650485, 0.8047378541243650485, 1.000000000000000000 ) ) 
 REPRESENTATION_ITEM ( '' )  );
#9863=ORIENTED_EDGE ( 'NONE', *, *, #1259, .F. ) ;
#9866=EDGE_LOOP ( 'NONE', ( #6615, #14968, #7592, #1024 ) ) ;
#9908=CIRCLE ( 'NONE', #3717, 9.999999999999980460 ) ;
#9909=CARTESIAN_POINT ( 'NONE',  ( -116.3391301858327296, -120.2076149402627294, 7.500000000000001776 ) ) ;
#9925=AXIS2_PLACEMENT_3D ( 'NONE', #10883, #15824, #2385 ) ;
#9950=VECTOR ( 'NONE', #4998, 1000.000000000000000 ) ;
#9956=PLANE ( 'NONE',  #4812 ) ;
#9981=VERTEX_POINT ( 'NONE', #9296 ) ;
#10002=CARTESIAN_POINT ( 'NONE',  ( -91.33974596215560382, -110.0591436588189396, -7.500000000000000000 ) ) ;
#10028=CARTESIAN_POINT ( 'NONE',  ( -91.33974596215558961, -105.7735026918962546, -7.500000000000000000 ) ) ;
#10074=VECTOR ( 'NONE', #5688, 1000.000000000000000 ) ;
#10077=EDGE_LOOP ( 'NONE', ( #26, #6556, #14624 ) ) ;
#10079=ORIENTED_EDGE ( 'NONE', *, *, #145, .F. ) ;
#10124=FACE_OUTER_BOUND ( 'NONE', #6774, .T. ) ;
#10136=CARTESIAN_POINT ( 'NONE',  ( -115.0000000000000142, -3.122502256758252770E-14, -7.500000000000000000 ) ) ;
#10151=CARTESIAN_POINT ( 'NONE',  ( -54.99999999999999289, -25.00000000000000000, 17.50000000000000000 ) ) ;
#10186=CARTESIAN_POINT ( 'NONE',  ( -115.0000000000000142, -10.00000000000000888, -7.500000000000000000 ) ) ;
#10187=DIRECTION ( 'NONE',  ( -1.000000000000000000, 0.000000000000000000, 0.000000000000000000 ) ) ;
#10210=VERTEX_POINT ( 'NONE', #7273 ) ;
#10213=VECTOR ( 'NONE', #3454, 1000.000000000000000 ) ;
#10227=CARTESIAN_POINT ( 'NONE',  ( -45.00000000000000000, 0.000000000000000000, 7.500000000000001776 ) ) ;
#10246=DIRECTION ( 'NONE',  ( -0.000000000000000000, -1.000000000000000000, -0.000000000000000000 ) ) ;
#10260=ORIENTED_EDGE ( 'NONE', *, *, #1684, .T. ) ;
#10265=AXIS2_PLACEMENT_3D ( 'NONE', #9573, #7081, #12066 ) ;
#10280=VERTEX_POINT ( 'NONE', #5814 ) ;
#10294=EDGE_CURVE ( 'NONE', #14193, #6058, #14604, .T. ) ;
#10298=DIRECTION ( 'NONE',  ( 0.000000000000000000, -1.000000000000000000, 0.000000000000000000 ) ) ;
#10302=ORIENTED_EDGE ( 'NONE', *, *, #10774, .T. ) ;
#10321=CARTESIAN_POINT ( 'NONE',  ( -116.3391301858327296, -120.2076149402627294, 7.500000000000001776 ) ) ;
#10324=ORIENTED_EDGE ( 'NONE', *, *, #10733, .F. ) ;
#10365=EDGE_CURVE ( 'NONE', #3476, #14971, #9284, .T. ) ;
#10376=DIRECTION ( 'NONE',  ( 0.000000000000000000, 1.000000000000000000, 0.000000000000000000 ) ) ;
#10411=PRODUCT_DEFINITION_SHAPE ( 'NONE', 'NONE',  #2153 ) ;
#10414=EDGE_CURVE ( 'NONE', #757, #5100, #14951, .T. ) ;
#10416=VECTOR ( 'NONE', #1290, 1000.000000000000000 ) ;
#10428=EDGE_CURVE ( 'NONE', #15817, #9981, #12789, .T. ) ;
#10464=LINE ( 'NONE', #9261, #9676 ) ;
#10495=CARTESIAN_POINT ( 'NONE',  ( -34.99999999999999289, -11.00000000000000178, 2.000000000000830447 ) ) ;
#10515=ADVANCED_FACE ( 'NONE', ( #7156 ), #13117, .T. ) ;
#10520=ORIENTED_EDGE ( 'NONE', *, *, #3648, .T. ) ;
#10525=CARTESIAN_POINT ( 'NONE',  ( -39.99999999999999289, -11.00000000000000178, 8.300651832549021947E-13 ) ) ;
#10540=ORIENTED_EDGE ( 'NONE', *, *, #8418, .T. ) ;
#10553=CARTESIAN_POINT ( 'NONE',  ( -39.99999999999999289, -11.00000000000000178, 2.500000000001739497 ) ) ;
#10560=DIRECTION ( 'NONE',  ( -0.000000000000000000, -0.000000000000000000, 1.000000000000000000 ) ) ;
#10569=CARTESIAN_POINT ( 'NONE',  ( -150.5560796608385203, -71.58493649053927754, 7.500000000000001776 ) ) ;
#10571=ADVANCED_FACE ( 'NONE', ( #4715 ), #13188, .T. ) ;
#10582=VECTOR ( 'NONE', #11573, 1000.000000000000000 ) ;
#10591=ADVANCED_FACE ( 'NONE', ( #4953 ), #4797, .T. ) ;
#10606=LINE ( 'NONE', #9459, #677 ) ;
#10607=ORIENTED_EDGE ( 'NONE', *, *, #2414, .F. ) ;
#10613=DIRECTION ( 'NONE',  ( -1.000000000000000000, 0.000000000000000000, 0.000000000000000000 ) ) ;
#10614=CARTESIAN_POINT ( 'NONE',  ( -91.33974596215560382, -110.0591436588189396, 7.500000000000001776 ) ) ;
#10625=CARTESIAN_POINT ( 'NONE',  ( -44.99999999999999289, -11.00000000000000178, -3.999999999999170885 ) ) ;
#10627=ORIENTED_EDGE ( 'NONE', *, *, #11721, .T. ) ;
#10631=ADVANCED_FACE ( 'NONE', ( #8683 ), #6257, .T. ) ;
#10643=DIRECTION ( 'NONE',  ( 0.000000000000000000, 1.000000000000000000, -0.000000000000000000 ) ) ;
#10650=ORIENTED_EDGE ( 'NONE', *, *, #8376, .F. ) ;
#10661=CARTESIAN_POINT ( 'NONE',  ( -124.9999999999999858, -115.2072594216369907, 17.50000000000000000 ) ) ;
#10664=ORIENTED_EDGE ( 'NONE', *, *, #5683, .F. ) ;
#10726=ORIENTED_EDGE ( 'NONE', *, *, #1072, .F. ) ;
#10731=CARTESIAN_POINT ( 'NONE',  ( -124.9999999999999716, -115.2072594216369623, -13.35786437626904721 ) ) ;
#10733=EDGE_CURVE ( 'NONE', #7722, #6759, #14970, .T. ) ;
#10774=EDGE_CURVE ( 'NONE', #2789, #10280, #6745, .T. ) ;
#10780=CIRCLE ( 'NONE', #14178, 9.999999999999994671 ) ;
#10795=ADVANCED_FACE ( 'NONE', ( #5443 ), #1477, .T. ) ;
#10799=VECTOR ( 'NONE', #6388, 1000.000000000000000 ) ;
#10808=ORIENTED_EDGE ( 'NONE', *, *, #2042, .F. ) ;
#10824=PLANE ( 'NONE',  #14332 ) ;
#10833=DIRECTION ( 'NONE',  ( -0.000000000000000000, -0.000000000000000000, -1.000000000000000000 ) ) ;
#10835=CARTESIAN_POINT ( 'NONE',  ( -91.33974596215560382, -110.0591436588189396, 17.50000000000000000 ) ) ;
#10842=EDGE_CURVE ( 'NONE', #11920, #4817, #12618, .T. ) ;
#10852=CARTESIAN_POINT ( 'NONE',  ( -90.00000000000000000, -35.00000000000000711, 17.50000000000000000 ) ) ;
#10858=CARTESIAN_POINT ( 'NONE',  ( -114.9999999999999716, -10.00000000000000888, 7.500000000000001776 ) ) ;
#10883=CARTESIAN_POINT ( 'NONE',  ( -45.00000000000000000, 0.000000000000000000, 17.50000000000000000 ) ) ;
#10885=CARTESIAN_POINT ( 'NONE',  ( -114.9999999999999858, -109.4337567297407219, 17.50000000000000000 ) ) ;
#10914=VECTOR ( 'NONE', #3091, 1000.000000000000000 ) ;
#10935=VERTEX_POINT ( 'NONE', #3101 ) ;
#10949=SURFACE_STYLE_FILL_AREA ( #14585 ) ;
#10962=ADVANCED_FACE ( 'NONE', ( #4393 ), #3172, .T. ) ;
#10963=CARTESIAN_POINT ( 'NONE',  ( -91.33974596215558961, -105.7735026918962546, 7.500000000000001776 ) ) ;
#10975=ORIENTED_EDGE ( 'NONE', *, *, #10733, .T. ) ;
#10990=CIRCLE ( 'NONE', #1175, 10.00000000000000000 ) ;
#11000=ORIENTED_EDGE ( 'NONE', *, *, #5683, .T. ) ;
#11005=CIRCLE ( 'NONE', #7664, 10.00000000000000000 ) ;
#11017=LINE ( 'NONE', #12209, #7973 ) ;
#11039=VECTOR ( 'NONE', #12037, 1000.000000000000000 ) ;
#11044=VERTEX_POINT ( 'NONE', #3804 ) ;
#11051=VECTOR ( 'NONE', #977, 1000.000000000000000 ) ;
#11053=CARTESIAN_POINT ( 'NONE',  ( -91.33974596215557540, -105.7735026918962689, 17.50000000000000000 ) ) ;
#11060=VECTOR ( 'NONE', #14098, 1000.000000000000000 ) ;
#11072=CARTESIAN_POINT ( 'NONE',  ( -124.9999999999999858, -115.2072594216369907, 17.50000000000000000 ) ) ;
#11078=( BOUNDED_CURVE ( )  B_SPLINE_CURVE ( 3, ( #7585, #1589, #15016, #11290 ),
 .UNSPECIFIED., .F., .F. ) 
 B_SPLINE_CURVE_WITH_KNOTS ( ( 4, 4 ),
 ( 1.570796326794896780, 3.141592653589793116 ),
 .UNSPECIFIED. ) 
 CURVE ( )  GEOMETRIC_REPRESENTATION_ITEM ( )  RATIONAL_B_SPLINE_CURVE ( ( 1.000000000000000000, 0.8047378541243650485, 0.8047378541243650485, 1.000000000000000000 ) ) 
 REPRESENTATION_ITEM ( '' )  );
#11089=EDGE_CURVE ( 'NONE', #11044, #3131, #9151, .T. ) ;
#11097=DIRECTION ( 'NONE',  ( -0.4999999999999966138, -0.8660254037844405950, 0.000000000000000000 ) ) ;
#11101=DIRECTION ( 'NONE',  ( 0.9999824063907752913, 0.005931855436079607087, 0.000000000000000000 ) ) ;
#11111=EDGE_CURVE ( 'NONE', #7180, #11920, #7458, .T. ) ;
#11117=VERTEX_POINT ( 'NONE', #12364 ) ;
#11136=ORIENTED_EDGE ( 'NONE', *, *, #6671, .T. ) ;
#11141=CARTESIAN_POINT ( 'NONE',  ( -94.99999999999994316, -103.6602540378444246, 17.50000000000000000 ) ) ;
#11186=ORIENTED_EDGE ( 'NONE', *, *, #12350, .T. ) ;
#11193=VERTEX_POINT ( 'NONE', #12676 ) ;
#11204=DIRECTION ( 'NONE',  ( 0.8660254037844407060, -0.4999999999999965028, 0.000000000000000000 ) ) ;
#11218=AXIS2_PLACEMENT_3D ( 'NONE', #14289, #11851, #798 ) ;
#11262=DIRECTION ( 'NONE',  ( -1.000000000000000000, 0.000000000000000000, 0.000000000000000000 ) ) ;
#11263=AXIS2_PLACEMENT_3D ( 'NONE', #12958, #14269, #14196 ) ;
#11266=CARTESIAN_POINT ( 'NONE',  ( -81.33974596215558961, -105.7735026918962404, -7.500000000000000000 ) ) ;
#11288=CARTESIAN_POINT ( 'NONE',  ( -90.00000000000000000, -95.00000000000000000, 17.50000000000000000 ) ) ;
#11290=CARTESIAN_POINT ( 'NONE',  ( -44.99999999999999289, -35.00000000000000000, -7.500000000000000000 ) ) ;
#11330=AXIS2_PLACEMENT_3D ( 'NONE', #5538, #1352, #1652 ) ;
#11352=EDGE_CURVE ( 'NONE', #9981, #1886, #10606, .T. ) ;
#11361=CARTESIAN_POINT ( 'NONE',  ( -49.14213562373094391, -4.142135623730951899, -17.49999999999999645 ) ) ;
#11367=CYLINDRICAL_SURFACE ( 'NONE', #3951, 10.00000000000000000 ) ;
#11406=CARTESIAN_POINT ( 'NONE',  ( -91.33974596215558961, -105.7735026918962404, 7.500000000000001776 ) ) ;
#11420=DIRECTION ( 'NONE',  ( 0.000000000000000000, 0.000000000000000000, -1.000000000000000000 ) ) ;
#11435=DIRECTION ( 'NONE',  ( 2.775557561562896479E-15, -1.000000000000000000, -0.000000000000000000 ) ) ;
#11443=DIRECTION ( 'NONE',  ( -0.8660254037844402619, 0.4999999999999973910, 0.000000000000000000 ) ) ;
#11464=LINE ( 'NONE', #13801, #3545 ) ;
#11488=ORIENTED_EDGE ( 'NONE', *, *, #979, .F. ) ;
#11500=SPHERICAL_SURFACE ( 'NONE', #7078, 10.00000000000000000 ) ;
#11504=DIRECTION ( 'NONE',  ( -0.9999824063907751803, -0.005931855436079011210, -0.000000000000000000 ) ) ;
#11509=ORIENTED_EDGE ( 'NONE', *, *, #6306, .T. ) ;
#11510=VECTOR ( 'NONE', #4405, 1000.000000000000000 ) ;
#11525=CIRCLE ( 'NONE', #7928, 9.999999999999994671 ) ;
#11530=VERTEX_POINT ( 'NONE', #14621 ) ;
#11531=ORIENTED_EDGE ( 'NONE', *, *, #15882, .T. ) ;
#11551=EDGE_CURVE ( 'NONE', #14039, #6759, #10990, .T. ) ;
#11556=AXIS2_PLACEMENT_3D ( 'NONE', #15379, #4302, #10298 ) ;
#11573=DIRECTION ( 'NONE',  ( 1.982541115402065110E-16, -1.000000000000000000, -0.000000000000000000 ) ) ;
#11575=COLOUR_RGB ( '', 0.09019608, 0.27058824, 0.51372549) ;
#11594=ORIENTED_EDGE ( 'NONE', *, *, #12143, .F. ) ;
#11607=ORIENTED_EDGE ( 'NONE', *, *, #5242, .F. ) ;
#11641=DIRECTION ( 'NONE',  ( 1.000000000000000000, -1.387778780781446464E-15, 0.000000000000000000 ) ) ;
#11644=VERTEX_POINT ( 'NONE', #253 ) ;
#11656=DIRECTION ( 'NONE',  ( 0.000000000000000000, 0.000000000000000000, -1.000000000000000000 ) ) ;
#11678=AXIS2_PLACEMENT_3D ( 'NONE', #13963, #8977, #13889 ) ;
#11697=DIRECTION ( 'NONE',  ( -0.8660254037844401509, 0.4999999999999973355, -0.000000000000000000 ) ) ;
#11710=DIRECTION ( 'NONE',  ( 0.000000000000000000, 0.000000000000000000, -1.000000000000000000 ) ) ;
#11721=EDGE_CURVE ( 'NONE', #11920, #13100, #13830, .T. ) ;
#11729=CIRCLE ( 'NONE', #13269, 9.999999999999994671 ) ;
#11733=DIRECTION ( 'NONE',  ( 1.000000000000000000, 0.000000000000000000, 0.000000000000000000 ) ) ;
#11739=EDGE_CURVE ( 'NONE', #9005, #5616, #11005, .T. ) ;
#11744=ADVANCED_FACE ( 'NONE', ( #8969 ), #7841, .F. ) ;
#11748=DIRECTION ( 'NONE',  ( 0.000000000000000000, 1.000000000000000000, -0.000000000000000000 ) ) ;
#11765=CIRCLE ( 'NONE', #12279, 10.00000000000000000 ) ;
#11768=DIRECTION ( 'NONE',  ( 0.8660254037844407060, -0.4999999999999966693, 0.000000000000000000 ) ) ;
#11781=ORIENTED_EDGE ( 'NONE', *, *, #12839, .F. ) ;
#11792=AXIS2_PLACEMENT_3D ( 'NONE', #212, #11420, #15151 ) ;
#11811=VECTOR ( 'NONE', #1344, 1000.000000000000000 ) ;
#11847=ORIENTED_EDGE ( 'NONE', *, *, #5435, .T. ) ;
#11851=DIRECTION ( 'NONE',  ( 0.8660254037844402619, -0.4999999999999973910, 0.000000000000000000 ) ) ;
#11872=DIRECTION ( 'NONE',  ( 0.000000000000000000, 0.000000000000000000, 1.000000000000000000 ) ) ;
#11873=CARTESIAN_POINT ( 'NONE',  ( -49.14213562373093680, -30.85786437626904899, 17.49999999999999645 ) ) ;
#11878=CYLINDRICAL_SURFACE ( 'NONE', #13799, 9.999999999999994671 ) ;
#11887=DIRECTION ( 'NONE',  ( -0.000000000000000000, -0.000000000000000000, -1.000000000000000000 ) ) ;
#11897=CARTESIAN_POINT ( 'NONE',  ( 0.000000000000000000, 0.000000000000000000, 0.000000000000000000 ) ) ;
#11901=ORIENTED_EDGE ( 'NONE', *, *, #11739, .F. ) ;
#11904=CARTESIAN_POINT ( 'NONE',  ( -99.99999999999998579, -25.00000000000000711, -17.50000000000000000 ) ) ;
#11905=VECTOR ( 'NONE', #14505, 1000.000000000000000 ) ;
#11914=DIRECTION ( 'NONE',  ( -0.9999824063907751803, -0.005931855436079011210, 0.000000000000000000 ) ) ;
#11919=ORIENTED_EDGE ( 'NONE', *, *, #1995, .F. ) ;
#11920=VERTEX_POINT ( 'NONE', #1763 ) ;
#11931=DIRECTION ( 'NONE',  ( -0.8660254037844402619, 0.4999999999999973355, 0.000000000000000000 ) ) ;
#11944=EDGE_CURVE ( 'NONE', #7180, #5811, #2735, .T. ) ;
#11960=EDGE_CURVE ( 'NONE', #7410, #757, #5646, .T. ) ;
#11972=DIRECTION ( 'NONE',  ( 0.000000000000000000, 0.000000000000000000, 1.000000000000000000 ) ) ;
#12005=CARTESIAN_POINT ( 'NONE',  ( -90.00000000000000000, -35.00000000000000711, 17.50000000000000000 ) ) ;
#12027=CARTESIAN_POINT ( 'NONE',  ( -116.3391301858327296, -120.2076149402627294, 17.50000000000000000 ) ) ;
#12028=DIRECTION ( 'NONE',  ( 1.000000000000000000, 0.000000000000000000, 0.000000000000000000 ) ) ;
#12029=CARTESIAN_POINT ( 'NONE',  ( -99.99999999999998579, -100.7735026918963115, 17.50000000000000000 ) ) ;
#12037=DIRECTION ( 'NONE',  ( 0.000000000000000000, 1.000000000000000000, -0.000000000000000000 ) ) ;
#12050=EDGE_CURVE ( 'NONE', #1886, #7410, #11765, .T. ) ;
#12062=CARTESIAN_POINT ( 'NONE',  ( -99.99999999999998579, -100.7735026918963115, 17.50000000000000000 ) ) ;
#12066=DIRECTION ( 'NONE',  ( 1.000000000000000000, 0.000000000000000000, -0.000000000000000000 ) ) ;
#12067=LINE ( 'NONE', #1083, #11905 ) ;
#12087=DIRECTION ( 'NONE',  ( -1.000000000000000000, 0.000000000000000000, 0.000000000000000000 ) ) ;
#12135=ORIENTED_EDGE ( 'NONE', *, *, #13824, .T. ) ;
#12143=EDGE_CURVE ( 'NONE', #5100, #2789, #14090, .T. ) ;
#12149=PRESENTATION_STYLE_ASSIGNMENT (( #4811 ) ) ;
#12176=CARTESIAN_POINT ( 'NONE',  ( -115.0000000000000142, -10.00000000000000888, -7.500000000000000000 ) ) ;
#12178=AXIS2_PLACEMENT_3D ( 'NONE', #8737, #1360, #3547 ) ;
#12209=CARTESIAN_POINT ( 'NONE',  ( -124.9999999999999716, -10.00000000000001066, -7.500000000000000000 ) ) ;
#12225=EDGE_CURVE ( 'NONE', #6165, #1597, #11525, .T. ) ;
#12234=EDGE_LOOP ( 'NONE', ( #10975, #8532, #2327, #14903 ) ) ;
#12238=PLANE ( 'NONE',  #9925 ) ;
#12240=CARTESIAN_POINT ( 'NONE',  ( -124.9999999999999858, -115.2072594216369907, -7.500000000000000000 ) ) ;
#12241=CARTESIAN_POINT ( 'NONE',  ( -99.99999999999998579, -10.00000000000000888, -17.50000000000000000 ) ) ;
#12244=CARTESIAN_POINT ( 'NONE',  ( -44.99999999999999289, -13.00000000000000178, -3.999999999999170885 ) ) ;
#12251=VECTOR ( 'NONE', #13475, 1000.000000000000000 ) ;
#12256=CARTESIAN_POINT ( 'NONE',  ( -90.00000000000000000, -94.99999999999995737, -13.35786437626905077 ) ) ;
#12268=DIRECTION ( 'NONE',  ( 0.000000000000000000, 0.000000000000000000, 1.000000000000000000 ) ) ;
#12279=AXIS2_PLACEMENT_3D ( 'NONE', #2314, #15752, #8475 ) ;
#12301=EDGE_CURVE ( 'NONE', #5616, #11530, #7147, .T. ) ;
#12307=( NAMED_UNIT ( * ) SI_UNIT ( $, .STERADIAN. ) SOLID_ANGLE_UNIT ( ) );
#12343=DIRECTION ( 'NONE',  ( 0.000000000000000000, 0.000000000000000000, 1.000000000000000000 ) ) ;
#12350=EDGE_CURVE ( 'NONE', #8889, #2808, #2224, .T. ) ;
#12364=CARTESIAN_POINT ( 'NONE',  ( -116.3391301858327296, -120.2076149402627294, -7.500000000000000000 ) ) ;
#12377=ORIENTED_EDGE ( 'NONE', *, *, #2334, .T. ) ;
#12391=ORIENTED_EDGE ( 'NONE', *, *, #5739, .T. ) ;
#12401=CARTESIAN_POINT ( 'NONE',  ( -91.33974596215557540, -105.7735026918962689, 7.500000000000001776 ) ) ;
#12405=CARTESIAN_POINT ( 'NONE',  ( -44.99999999999999289, -35.00000000000000711, 7.500000000000001776 ) ) ;
#12509=CARTESIAN_POINT ( 'NONE',  ( -44.99999999999999289, -35.00000000000000000, 7.500000000000001776 ) ) ;
#12535=ORIENTED_EDGE ( 'NONE', *, *, #2334, .F. ) ;
#12542=EDGE_CURVE ( 'NONE', #10210, #8136, #5218, .T. ) ;
#12549=CARTESIAN_POINT ( 'NONE',  ( -45.00000000000000711, -2.452104961800526543E-15, 13.35786437626905077 ) ) ;
#12555=CARTESIAN_POINT ( 'NONE',  ( -34.99999999999999289, -11.00000000000000178, -1.999999999999170441 ) ) ;
#12561=DIRECTION ( 'NONE',  ( -0.005931855436078210635, 0.9999824063907751803, 0.000000000000000000 ) ) ;
#12589=AXIS2_PLACEMENT_3D ( 'NONE', #2932, #5374, #6911 ) ;
#12601=VECTOR ( 'NONE', #2632, 1000.000000000000000 ) ;
#12611=VECTOR ( 'NONE', #4220, 1000.000000000000000 ) ;
#12616=FILL_AREA_STYLE ('',( #5198 ) ) ;
#12618=LINE ( 'NONE', #1560, #12611 ) ;
#12629=CARTESIAN_POINT ( 'NONE',  ( -39.99999999999999289, -13.00000000000000178, 2.500000000001739497 ) ) ;
#12660=CARTESIAN_POINT ( 'NONE',  ( -91.33974596215560382, -110.0591436588189396, -7.500000000000001776 ) ) ;
#12676=CARTESIAN_POINT ( 'NONE',  ( -124.9999999999999858, -115.2072594216369907, -7.500000000000000000 ) ) ;
#12677=VECTOR ( 'NONE', #5946, 1000.000000000000000 ) ;
#12689=( LENGTH_UNIT ( ) NAMED_UNIT ( * ) SI_UNIT ( .MILLI., .METRE. ) );
#12706=CARTESIAN_POINT ( 'NONE',  ( -91.33974596215558961, -105.7735026918962262, -7.500000000000000000 ) ) ;
#12733=ORIENTED_EDGE ( 'NONE', *, *, #12143, .T. ) ;
#12754=AXIS2_PLACEMENT_3D ( 'NONE', #10569, #4245, #5466 ) ;
#12757=ORIENTED_EDGE ( 'NONE', *, *, #3164, .F. ) ;
#12769=VERTEX_POINT ( 'NONE', #350 ) ;
#12774=APPLICATION_CONTEXT ( 'automotive_design' ) ;
#12778=DIRECTION ( 'NONE',  ( 1.734723475976810299E-16, -1.000000000000000000, 0.000000000000000000 ) ) ;
#12780=AXIS2_PLACEMENT_3D ( 'NONE', #12660, #1529, #15100 ) ;
#12789=LINE ( 'NONE', #1276, #6673 ) ;
#12839=EDGE_CURVE ( 'NONE', #2808, #8889, #13007, .T. ) ;
#12847=LINE ( 'NONE', #13002, #10914 ) ;
#12855=AXIS2_PLACEMENT_3D ( 'NONE', #6694, #9042, #4341 ) ;
#12861=STYLED_ITEM ( 'NONE', ( #12149 ), #3386 ) ;
#12874=ORIENTED_EDGE ( 'NONE', *, *, #13355, .T. ) ;
#12882=AXIS2_PLACEMENT_3D ( 'NONE', #10858, #7076, #3116 ) ;
#12885=CARTESIAN_POINT ( 'NONE',  ( -113.6871902368262965, -110.1917077999038099, -17.50000000000000000 ) ) ;
#12892=ADVANCED_FACE ( 'NONE', ( #5901 ), #4380, .F. ) ;
#12920=EDGE_LOOP ( 'NONE', ( #11781, #7488 ) ) ;
#12944=EDGE_CURVE ( 'NONE', #3371, #11193, #4924, .T. ) ;
#12949=ORIENTED_EDGE ( 'NONE', *, *, #11111, .F. ) ;
#12954=DIRECTION ( 'NONE',  ( 0.005931855436079607087, -0.9999824063907751803, 0.000000000000000000 ) ) ;
#12958=CARTESIAN_POINT ( 'NONE',  ( -39.99999999999999289, -11.00000000000000178, 8.300651832549021947E-13 ) ) ;
#12971=ORIENTED_EDGE ( 'NONE', *, *, #14506, .T. ) ;
#13001=ADVANCED_FACE ( 'NONE', ( #7521 ), #7206, .T. ) ;
#13002=CARTESIAN_POINT ( 'NONE',  ( -81.33974596215558961, -99.99999999999995737, -7.500000000000000000 ) ) ;
#13007=CIRCLE ( 'NONE', #9191, 2.500000000000909495 ) ;
#13012=DIRECTION ( 'NONE',  ( 1.000000000000000000, 0.000000000000000000, 0.000000000000000000 ) ) ;
#13054=ORIENTED_EDGE ( 'NONE', *, *, #15417, .T. ) ;
#13058=VECTOR ( 'NONE', #8844, 1000.000000000000000 ) ;
#13060=DIRECTION ( 'NONE',  ( 0.4999999999999960032, 0.8660254037844409281, 0.000000000000000000 ) ) ;
#13071=PLANE ( 'NONE',  #9159 ) ;
#13077=CARTESIAN_POINT ( 'NONE',  ( -124.9999999999999716, -10.00000000000001066, 17.50000000000000000 ) ) ;
#13085=DIRECTION ( 'NONE',  ( 0.000000000000000000, 1.000000000000000000, 0.000000000000000000 ) ) ;
#13089=LINE ( 'NONE', #8345, #582 ) ;
#13097=EDGE_CURVE ( 'NONE', #1597, #13901, #80, .T. ) ;
#13100=VERTEX_POINT ( 'NONE', #1200 ) ;
#13108=LINE ( 'NONE', #6752, #3105 ) ;
#13114=AXIS2_PLACEMENT_3D ( 'NONE', #1959, #11887, #9482 ) ;
#13116=ORIENTED_EDGE ( 'NONE', *, *, #3425, .T. ) ;
#13117=CYLINDRICAL_SURFACE ( 'NONE', #9543, 9.999999999999992895 ) ;
#13121=CARTESIAN_POINT ( 'NONE',  ( -94.14213562373093680, -30.85786437626904899, -17.49999999999999645 ) ) ;
#13128=DIRECTION ( 'NONE',  ( -1.319090325525611458E-16, -1.000000000000000000, 0.000000000000000000 ) ) ;
#13138=AXIS2_PLACEMENT_3D ( 'NONE', #13584, #6091, #8601 ) ;
#13145=FACE_OUTER_BOUND ( 'NONE', #2293, .T. ) ;
#13155=VERTEX_POINT ( 'NONE', #15273 ) ;
#13159=EDGE_LOOP ( 'NONE', ( #13116, #1614, #6280, #9293 ) ) ;
#13182=PLANE ( 'NONE',  #2258 ) ;
#13188=CYLINDRICAL_SURFACE ( 'NONE', #12882, 9.999999999999994671 ) ;
#13207=ORIENTED_EDGE ( 'NONE', *, *, #4109, .F. ) ;
#13208=ORIENTED_EDGE ( 'NONE', *, *, #7446, .T. ) ;
#13225=CIRCLE ( 'NONE', #8613, 9.999999999999994671 ) ;
#13239=CARTESIAN_POINT ( 'NONE',  ( -44.99999999999999289, -35.00000000000000000, 7.500000000000001776 ) ) ;
#13269=AXIS2_PLACEMENT_3D ( 'NONE', #12706, #7654, #1498 ) ;
#13310=CARTESIAN_POINT ( 'NONE',  ( -116.3984487401935155, -110.2077908763549914, -7.500000000000000000 ) ) ;
#13321=DIRECTION ( 'NONE',  ( -0.000000000000000000, -0.000000000000000000, -1.000000000000000000 ) ) ;
#13332=VECTOR ( 'NONE', #765, 1000.000000000000000 ) ;
#13340=VECTOR ( 'NONE', #11697, 1000.000000000000000 ) ;
#13345=ADVANCED_FACE ( 'NONE', ( #13145 ), #722, .T. ) ;
#13355=EDGE_CURVE ( 'NONE', #11193, #7310, #9058, .T. ) ;
#13363=SURFACE_SIDE_STYLE ('',( #10949 ) ) ;
#13405=CARTESIAN_POINT ( 'NONE',  ( -36.99999999999999289, -11.00000000000000178, 2.000000000000830891 ) ) ;
#13428=CARTESIAN_POINT ( 'NONE',  ( -114.9999999999999716, -10.00000000000000888, -17.50000000000000000 ) ) ;
#13429=PLANE ( 'NONE',  #10265 ) ;
#13446=CARTESIAN_POINT ( 'NONE',  ( -44.99999999999999289, -11.00000000000000178, -3.999999999999170885 ) ) ;
#13462=CIRCLE ( 'NONE', #12178, 9.999999999999994671 ) ;
#13467=CARTESIAN_POINT ( 'NONE',  ( -115.0000000000000142, -25.00000000000001066, -17.50000000000000000 ) ) ;
#13475=DIRECTION ( 'NONE',  ( -0.000000000000000000, -1.000000000000000000, -0.000000000000000000 ) ) ;
#13481=ADVANCED_FACE ( 'NONE', ( #1028, #5962 ), #12238, .F. ) ;
#13505=LINE ( 'NONE', #2442, #8350 ) ;
#13509=( LENGTH_UNIT ( ) NAMED_UNIT ( * ) SI_UNIT ( .MILLI., .METRE. ) );
#13528=LINE ( 'NONE', #13446, #3931 ) ;
#13529=CARTESIAN_POINT ( 'NONE',  ( -115.2406606923553056, -116.0588903632565092, 17.50000000000000711 ) ) ;
#13554=CARTESIAN_POINT ( 'NONE',  ( -114.9999999999999716, -10.00000000000001243, -7.500000000000000000 ) ) ;
#13560=ORIENTED_EDGE ( 'NONE', *, *, #5447, .T. ) ;
#13583=EDGE_LOOP ( 'NONE', ( #11594, #11919, #6623, #9765 ) ) ;
#13584=CARTESIAN_POINT ( 'NONE',  ( -91.33974596215558961, -105.7735026918962404, 17.50000000000000000 ) ) ;
#13594=VECTOR ( 'NONE', #13128, 1000.000000000000000 ) ;
#13597=CARTESIAN_POINT ( 'NONE',  ( -55.00000000000000000, -1.982541115402065307E-15, -7.500000000000000000 ) ) ;
#13616=PLANE ( 'NONE',  #6384 ) ;
#13642=DIRECTION ( 'NONE',  ( 0.000000000000000000, 1.000000000000000000, 0.000000000000000000 ) ) ;
#13675=ADVANCED_FACE ( 'NONE', ( #549 ), #4487, .T. ) ;
#13676=FACE_OUTER_BOUND ( 'NONE', #9866, .T. ) ;
#13695=DIRECTION ( 'NONE',  ( 0.9999824063907752913, 0.005931855436078211502, -0.000000000000000000 ) ) ;
#13748=DIRECTION ( 'NONE',  ( 1.000000000000000000, 1.734723475976808080E-16, 0.000000000000000000 ) ) ;
#13763=CARTESIAN_POINT ( 'NONE',  ( -34.99999999999999289, -11.00000000000000178, -1.999999999999170441 ) ) ;
#13779=CARTESIAN_POINT ( 'NONE',  ( -45.00000000000000000, -10.00000000000000000, -7.500000000000000000 ) ) ;
#13780=EDGE_CURVE ( 'NONE', #11117, #4817, #5312, .T. ) ;
#13786=DIRECTION ( 'NONE',  ( 0.000000000000000000, 1.000000000000000000, -0.000000000000000000 ) ) ;
#13791=VECTOR ( 'NONE', #7393, 1000.000000000000000 ) ;
#13799=AXIS2_PLACEMENT_3D ( 'NONE', #8431, #8192, #10613 ) ;
#13801=CARTESIAN_POINT ( 'NONE',  ( -115.0000000000000142, -10.00000000000000888, -17.50000000000000000 ) ) ;
#13802=EDGE_CURVE ( 'NONE', #3371, #658, #14198, .T. ) ;
#13807=CARTESIAN_POINT ( 'NONE',  ( -44.99999999999999289, -11.00000000000000178, 4.000000000000831335 ) ) ;
#13809=ORIENTED_EDGE ( 'NONE', *, *, #15882, .F. ) ;
#13823=EDGE_CURVE ( 'NONE', #11644, #1547, #9167, .T. ) ;
#13824=EDGE_CURVE ( 'NONE', #14832, #10935, #9812, .T. ) ;
#13829=VERTEX_POINT ( 'NONE', #7163 ) ;
#13830=CIRCLE ( 'NONE', #12780, 9.999999999999994671 ) ;
#13834=EDGE_LOOP ( 'NONE', ( #930, #13976, #306, #5918 ) ) ;
#13840=VECTOR ( 'NONE', #9181, 1000.000000000000000 ) ;
#13844=FACE_OUTER_BOUND ( 'NONE', #3757, .T. ) ;
#13857=EDGE_LOOP ( 'NONE', ( #14043, #6180, #2962, #11509 ) ) ;
#13858=ORIENTED_EDGE ( 'NONE', *, *, #3425, .F. ) ;
#13860=ORIENTED_EDGE ( 'NONE', *, *, #1610, .F. ) ;
#13880=DIRECTION ( 'NONE',  ( 0.000000000000000000, 0.000000000000000000, -1.000000000000000000 ) ) ;
#13889=DIRECTION ( 'NONE',  ( 0.000000000000000000, 0.000000000000000000, -1.000000000000000000 ) ) ;
#13901=VERTEX_POINT ( 'NONE', #12062 ) ;
#13918=CARTESIAN_POINT ( 'NONE',  ( -55.00000000000000000, -9.999999999999996447, -17.50000000000000000 ) ) ;
#13934=ORIENTED_EDGE ( 'NONE', *, *, #14524, .T. ) ;
#13935=ORIENTED_EDGE ( 'NONE', *, *, #1995, .T. ) ;
#13942=DIRECTION ( 'NONE',  ( 0.000000000000000000, 0.000000000000000000, 1.000000000000000000 ) ) ;
#13953=EDGE_LOOP ( 'NONE', ( #13934, #11488, #224, #12949 ) ) ;
#13963=CARTESIAN_POINT ( 'NONE',  ( -39.99999999999999289, -11.00000000000000178, 8.300651832549021947E-13 ) ) ;
#13976=ORIENTED_EDGE ( 'NONE', *, *, #14448, .T. ) ;
#14008=ADVANCED_FACE ( 'NONE', ( #13676 ), #7479, .T. ) ;
#14014=EDGE_LOOP ( 'NONE', ( #1372, #8910, #12757, #5807, #7368, #4676 ) ) ;
#14015=CARTESIAN_POINT ( 'NONE',  ( -45.00000000000000000, 0.000000000000000000, 17.50000000000000000 ) ) ;
#14039=VERTEX_POINT ( 'NONE', #10136 ) ;
#14043=ORIENTED_EDGE ( 'NONE', *, *, #3664, .T. ) ;
#14063=EDGE_LOOP ( 'NONE', ( #14493, #13935, #1314, #3495 ) ) ;
#14068=AXIS2_PLACEMENT_3D ( 'NONE', #14336, #15855, #8050 ) ;
#14083=ORIENTED_EDGE ( 'NONE', *, *, #1181, .T. ) ;
#14090=( BOUNDED_CURVE ( )  B_SPLINE_CURVE ( 3, ( #4085, #15008, #11361, #5221 ),
 .UNSPECIFIED., .F., .F. ) 
 B_SPLINE_CURVE_WITH_KNOTS ( ( 4, 4 ),
 ( 0.000000000000000000, 1.570796326794896558 ),
 .UNSPECIFIED. ) 
 CURVE ( )  GEOMETRIC_REPRESENTATION_ITEM ( )  RATIONAL_B_SPLINE_CURVE ( ( 1.000000000000000000, 0.8047378541243649375, 0.8047378541243649375, 1.000000000000000000 ) ) 
 REPRESENTATION_ITEM ( '' )  );
#14091=AXIS2_PLACEMENT_3D ( 'NONE', #5145, #14925, #9739 ) ;
#14096=CARTESIAN_POINT ( 'NONE',  ( -124.9999999999999716, -10.00000000000001066, 17.50000000000000000 ) ) ;
#14098=DIRECTION ( 'NONE',  ( -1.000000000000000000, -0.000000000000000000, -0.000000000000000000 ) ) ;
#14110=AXIS2_PLACEMENT_3D ( 'NONE', #1508, #13695, #12561 ) ;
#14120=CARTESIAN_POINT ( 'NONE',  ( -44.99999999999999289, -13.00000000000000178, -3.999999999999170885 ) ) ;
#14130=CARTESIAN_POINT ( 'NONE',  ( -91.33974596215558961, -105.7735026918962404, -7.500000000000001776 ) ) ;
#14149=ORIENTED_EDGE ( 'NONE', *, *, #7687, .T. ) ;
#14178=AXIS2_PLACEMENT_3D ( 'NONE', #10028, #7695, #10187 ) ;
#14188=CARTESIAN_POINT ( 'NONE',  ( -90.00000000000000000, -95.00000000000000000, -7.500000000000000000 ) ) ;
#14193=VERTEX_POINT ( 'NONE', #6820 ) ;
#14196=DIRECTION ( 'NONE',  ( 0.000000000000000000, 0.000000000000000000, 1.000000000000000000 ) ) ;
#14197=( BOUNDED_CURVE ( )  B_SPLINE_CURVE ( 3, ( #8031, #1858, #665, #12029 ),
 .UNSPECIFIED., .F., .F. ) 
 B_SPLINE_CURVE_WITH_KNOTS ( ( 4, 4 ),
 ( 3.141592653589793116, 4.712388980384691450 ),
 .UNSPECIFIED. ) 
 CURVE ( )  GEOMETRIC_REPRESENTATION_ITEM ( )  RATIONAL_B_SPLINE_CURVE ( ( 1.000000000000000000, 0.8047378541243646044, 0.8047378541243646044, 1.000000000000000000 ) ) 
 REPRESENTATION_ITEM ( '' )  );
#14198=LINE ( 'NONE', #3195, #6067 ) ;
#14204=DIRECTION ( 'NONE',  ( 0.000000000000000000, -1.000000000000000000, 0.000000000000000000 ) ) ;
#14208=CARTESIAN_POINT ( 'NONE',  ( -36.99999999999999289, -11.00000000000000178, 4.000000000000832223 ) ) ;
#14221=CARTESIAN_POINT ( 'NONE',  ( -34.99999999999999289, -11.00000000000000178, 2.000000000000830447 ) ) ;
#14241=CARTESIAN_POINT ( 'NONE',  ( -91.33974596215557540, -99.99999999999995737, 17.50000000000000000 ) ) ;
#14248=SURFACE_STYLE_USAGE ( .BOTH. , #15621 ) ;
#14265=ORIENTED_EDGE ( 'NONE', *, *, #13097, .T. ) ;
#14269=DIRECTION ( 'NONE',  ( 0.000000000000000000, 1.000000000000000000, 0.000000000000000000 ) ) ;
#14289=CARTESIAN_POINT ( 'NONE',  ( -120.0000000000000142, -106.5470053837925946, -7.500000000000000000 ) ) ;
#14304=ORIENTED_EDGE ( 'NONE', *, *, #1060, .T. ) ;
#14318=FACE_OUTER_BOUND ( 'NONE', #2906, .T. ) ;
#14332=AXIS2_PLACEMENT_3D ( 'NONE', #13077, #5810, #811 ) ;
#14336=CARTESIAN_POINT ( 'NONE',  ( -36.99999999999999289, -13.00000000000000178, 2.000000000000830891 ) ) ;
#14344=ORIENTED_EDGE ( 'NONE', *, *, #11089, .T. ) ;
#14370=AXIS2_PLACEMENT_3D ( 'NONE', #10963, #15906, #8557 ) ;
#14407=AXIS2_PLACEMENT_3D ( 'NONE', #9200, #14204, #3127 ) ;
#14408=ADVANCED_FACE ( 'NONE', ( #4691 ), #11878, .T. ) ;
#14420=VERTEX_POINT ( 'NONE', #4535 ) ;
#14423=AXIS2_PLACEMENT_3D ( 'NONE', #15311, #12778, #4146 ) ;
#14440=DIRECTION ( 'NONE',  ( -0.005931855436079011210, 0.9999824063907751803, 0.000000000000000000 ) ) ;
#14448=EDGE_CURVE ( 'NONE', #13155, #9599, #15341, .T. ) ;
#14464=VERTEX_POINT ( 'NONE', #15262 ) ;
#14480=SHAPE_REPRESENTATION_RELATIONSHIP ( 'NONE' , 'NONE' ,  #396, #6973 ) ;
#14493=ORIENTED_EDGE ( 'NONE', *, *, #5242, .T. ) ;
#14505=DIRECTION ( 'NONE',  ( 0.8660254037844401509, -0.4999999999999973355, 0.000000000000000000 ) ) ;
#14506=EDGE_CURVE ( 'NONE', #2790, #10935, #4073, .T. ) ;
#14515=ORIENTED_EDGE ( 'NONE', *, *, #8862, .T. ) ;
#14524=EDGE_CURVE ( 'NONE', #7180, #8026, #11729, .T. ) ;
#14526=DIRECTION ( 'NONE',  ( 0.8660254037844401509, -0.4999999999999973355, 0.000000000000000000 ) ) ;
#14552=CARTESIAN_POINT ( 'NONE',  ( -90.00000000000000000, -95.00000000000000000, 17.50000000000000000 ) ) ;
#14576=EDGE_CURVE ( 'NONE', #5972, #11644, #10464, .T. ) ;
#14578=MECHANICAL_DESIGN_GEOMETRIC_PRESENTATION_REPRESENTATION('',(#3998),#9673);
#14585=FILL_AREA_STYLE ('',( #6106 ) ) ;
#14604=( BOUNDED_CURVE ( )  B_SPLINE_CURVE ( 3, ( #6139, #14703, #12256, #4599 ),
 .UNSPECIFIED., .F., .F. ) 
 B_SPLINE_CURVE_WITH_KNOTS ( ( 4, 4 ),
 ( 1.570796326794896558, 3.141592653589793116 ),
 .UNSPECIFIED. ) 
 CURVE ( )  GEOMETRIC_REPRESENTATION_ITEM ( )  RATIONAL_B_SPLINE_CURVE ( ( 1.000000000000000000, 0.8047378541243649375, 0.8047378541243649375, 1.000000000000000000 ) ) 
 REPRESENTATION_ITEM ( '' )  );
#14606=VECTOR ( 'NONE', #394, 1000.000000000000000 ) ;
#14614=ORIENTED_EDGE ( 'NONE', *, *, #2414, .T. ) ;
#14615=LINE ( 'NONE', #4675, #10213 ) ;
#14621=CARTESIAN_POINT ( 'NONE',  ( -91.28042740779480368, -120.0589677227266918, 7.500000000000001776 ) ) ;
#14624=ORIENTED_EDGE ( 'NONE', *, *, #5507, .F. ) ;
#14689=DIRECTION ( 'NONE',  ( 0.000000000000000000, 1.000000000000000000, 0.000000000000000000 ) ) ;
#14695=ADVANCED_FACE ( 'NONE', ( #15398, #2345 ), #4322, .T. ) ;
#14703=CARTESIAN_POINT ( 'NONE',  ( -94.14213562373093680, -97.39146311738100792, -17.50000000000000000 ) ) ;
#14706=ORIENTED_EDGE ( 'NONE', *, *, #8108, .T. ) ;
#14718=LINE ( 'NONE', #5095, #10416 ) ;
#14722=ORIENTED_EDGE ( 'NONE', *, *, #1114, .T. ) ;
#14745=EDGE_CURVE ( 'NONE', #5972, #9599, #1541, .T. ) ;
#14765=CARTESIAN_POINT ( 'NONE',  ( -124.9999999999999716, -115.2072594216369339, 13.35786437626904366 ) ) ;
#14768=LINE ( 'NONE', #12244, #8870 ) ;
#14784=FACE_OUTER_BOUND ( 'NONE', #15544, .T. ) ;
#14820=VECTOR ( 'NONE', #9301, 1000.000000000000000 ) ;
#14832=VERTEX_POINT ( 'NONE', #6793 ) ;
#14892=DIRECTION ( 'NONE',  ( 0.000000000000000000, 0.000000000000000000, 1.000000000000000000 ) ) ;
#14903=ORIENTED_EDGE ( 'NONE', *, *, #6240, .F. ) ;
#14925=DIRECTION ( 'NONE',  ( 1.000000000000000000, 1.541976423090495140E-16, -0.000000000000000000 ) ) ;
#14948=EDGE_LOOP ( 'NONE', ( #3434, #10079, #3802, #12971 ) ) ;
#14951=LINE ( 'NONE', #14015, #9035 ) ;
#14963=CARTESIAN_POINT ( 'NONE',  ( -90.00000000000000000, -95.00000000000000000, 7.500000000000001776 ) ) ;
#14968=ORIENTED_EDGE ( 'NONE', *, *, #2589, .T. ) ;
#14970=CIRCLE ( 'NONE', #2308, 9.999999999999994671 ) ;
#14971=VERTEX_POINT ( 'NONE', #3534 ) ;
#14978=SHAPE_DEFINITION_REPRESENTATION ( #10411, #396 ) ;
#14981=LINE ( 'NONE', #9804, #15718 ) ;
#15008=CARTESIAN_POINT ( 'NONE',  ( -45.00000000000000711, -1.734723475976807094E-15, -13.35786437626904721 ) ) ;
#15016=CARTESIAN_POINT ( 'NONE',  ( -44.99999999999997868, -34.99999999999999289, -13.35786437626904544 ) ) ;
#15020=VERTEX_POINT ( 'NONE', #7198 ) ;
#15031=ADVANCED_FACE ( 'NONE', ( #8491 ), #10824, .F. ) ;
#15037=CYLINDRICAL_SURFACE ( 'NONE', #7089, 9.999999999999994671 ) ;
#15062=ORIENTED_EDGE ( 'NONE', *, *, #9686, .T. ) ;
#15075=EDGE_CURVE ( 'NONE', #12769, #13829, #14615, .T. ) ;
#15094=EDGE_LOOP ( 'NONE', ( #5817, #13809, #3957, #718 ) ) ;
#15100=DIRECTION ( 'NONE',  ( 1.000000000000000000, -1.387778780781446464E-15, 0.000000000000000000 ) ) ;
#15105=CARTESIAN_POINT ( 'NONE',  ( -44.99999999999999289, -13.00000000000000178, 4.000000000000831335 ) ) ;
#15110=LINE ( 'NONE', #14963, #8474 ) ;
#15122=ORIENTED_EDGE ( 'NONE', *, *, #4312, .T. ) ;
#15151=DIRECTION ( 'NONE',  ( -1.000000000000000000, 0.000000000000000000, -0.000000000000000000 ) ) ;
#15153=DIRECTION ( 'NONE',  ( -1.000000000000000000, 0.000000000000000000, 0.000000000000000000 ) ) ;
#15173=LINE ( 'NONE', #1587, #2033 ) ;
#15186=EDGE_LOOP ( 'NONE', ( #10260, #344, #5579, #7577, #3417, #4206 ) ) ;
#15234=EDGE_CURVE ( 'NONE', #2790, #14420, #7123, .T. ) ;
#15258=PLANE ( 'NONE',  #12855 ) ;
#15262=CARTESIAN_POINT ( 'NONE',  ( -44.99999999999999289, -35.00000000000000000, -7.500000000000000000 ) ) ;
#15273=CARTESIAN_POINT ( 'NONE',  ( -44.99999999999999289, -13.00000000000000178, -3.999999999999170885 ) ) ;
#15311=CARTESIAN_POINT ( 'NONE',  ( -115.0000000000000142, -10.00000000000000888, 7.500000000000001776 ) ) ;
#15320=CARTESIAN_POINT ( 'NONE',  ( -81.33974596215558961, -105.7735026918962404, 7.500000000000001776 ) ) ;
#15336=VECTOR ( 'NONE', #2613, 1000.000000000000000 ) ;
#15339=DIRECTION ( 'NONE',  ( 0.000000000000000000, 1.000000000000000000, -0.000000000000000000 ) ) ;
#15341=LINE ( 'NONE', #14120, #15883 ) ;
#15343=EDGE_LOOP ( 'NONE', ( #72, #7978, #5273, #6032 ) ) ;
#15347=EDGE_CURVE ( 'NONE', #1547, #14832, #559, .T. ) ;
#15379=CARTESIAN_POINT ( 'NONE',  ( -115.0000000000000142, -25.00000000000001066, 7.500000000000001776 ) ) ;
#15397=LINE ( 'NONE', #10625, #11060 ) ;
#15398=FACE_OUTER_BOUND ( 'NONE', #14014, .T. ) ;
#15402=DIRECTION ( 'NONE',  ( -0.000000000000000000, -0.000000000000000000, -1.000000000000000000 ) ) ;
#15417=EDGE_CURVE ( 'NONE', #11644, #6256, #6534, .T. ) ;
#15418=CARTESIAN_POINT ( 'NONE',  ( -124.9999999999999716, -10.00000000000001066, -7.500000000000000000 ) ) ;
#15421=DIRECTION ( 'NONE',  ( 0.000000000000000000, 0.000000000000000000, -1.000000000000000000 ) ) ;
#15430=( BOUNDED_CURVE ( )  B_SPLINE_CURVE ( 3, ( #1570, #1496, #12549, #10227 ),
 .UNSPECIFIED., .F., .F. ) 
 B_SPLINE_CURVE_WITH_KNOTS ( ( 4, 4 ),
 ( 1.570796326794896780, 3.141592653589793116 ),
 .UNSPECIFIED. ) 
 CURVE ( )  GEOMETRIC_REPRESENTATION_ITEM ( )  RATIONAL_B_SPLINE_CURVE ( ( 1.000000000000000000, 0.8047378541243650485, 0.8047378541243650485, 1.000000000000000000 ) ) 
 REPRESENTATION_ITEM ( '' )  );
#15437=AXIS2_PLACEMENT_3D ( 'NONE', #13405, #9617, #1129 ) ;
#15464=CIRCLE ( 'NONE', #14423, 9.999999999999994671 ) ;
#15480=LINE ( 'NONE', #683, #13332 ) ;
#15496=CARTESIAN_POINT ( 'NONE',  ( -115.2406606923551919, -116.0588903632565518, -17.49999999999999645 ) ) ;
#15513=CARTESIAN_POINT ( 'NONE',  ( -45.00000000000000000, 0.000000000000000000, 7.500000000000001776 ) ) ;
#15521=CARTESIAN_POINT ( 'NONE',  ( -55.00000000000000000, -10.00000000000000178, -17.50000000000000000 ) ) ;
#15544=EDGE_LOOP ( 'NONE', ( #15122, #206, #11607, #14149 ) ) ;
#15556=DIRECTION ( 'NONE',  ( -0.000000000000000000, -1.000000000000000000, -0.000000000000000000 ) ) ;
#15562=CARTESIAN_POINT ( 'NONE',  ( -90.00000000000000000, -35.00000000000000711, 7.500000000000001776 ) ) ;
#15577=CARTESIAN_POINT ( 'NONE',  ( -81.33974596215560382, -110.0591436588189538, 7.500000000000001776 ) ) ;
#15578=ADVANCED_FACE ( 'NONE', ( #8703 ), #1090, .T. ) ;
#15621=SURFACE_SIDE_STYLE ('',( #7797 ) ) ;
#15641=CARTESIAN_POINT ( 'NONE',  ( -91.28042740779480368, -120.0589677227266918, 17.50000000000000000 ) ) ;
#15665=ORIENTED_EDGE ( 'NONE', *, *, #1640, .T. ) ;
#15666=AXIS2_PLACEMENT_3D ( 'NONE', #9638, #11101, #3736 ) ;
#15671=VECTOR ( 'NONE', #14526, 1000.000000000000000 ) ;
#15677=CARTESIAN_POINT ( 'NONE',  ( -115.0000000000000142, -3.122502256758252770E-14, 17.50000000000000000 ) ) ;
#15689=ORIENTED_EDGE ( 'NONE', *, *, #1114, .F. ) ;
#15701=AXIS2_PLACEMENT_3D ( 'NONE', #6513, #1500, #6439 ) ;
#15702=CARTESIAN_POINT ( 'NONE',  ( -90.00000000000000000, -35.00000000000000711, -7.500000000000000000 ) ) ;
#15718=VECTOR ( 'NONE', #8838, 1000.000000000000000 ) ;
#15723=MECHANICAL_DESIGN_GEOMETRIC_PRESENTATION_REPRESENTATION('',(#12861),#4088);
#15739=LINE ( 'NONE', #1013, #12677 ) ;
#15752=DIRECTION ( 'NONE',  ( -1.000000000000000000, 0.000000000000000000, 0.000000000000000000 ) ) ;
#15764=EDGE_CURVE ( 'NONE', #1547, #2790, #5215, .T. ) ;
#15785=CARTESIAN_POINT ( 'NONE',  ( -90.00000000000000000, -35.00000000000000711, 7.500000000000001776 ) ) ;
#15792=DIRECTION ( 'NONE',  ( -1.000000000000000000, 0.000000000000000000, 0.000000000000000000 ) ) ;
#15795=VERTEX_POINT ( 'NONE', #10321 ) ;
#15817=VERTEX_POINT ( 'NONE', #10151 ) ;
#15824=DIRECTION ( 'NONE',  ( -1.000000000000000000, -1.982541115402065110E-16, 0.000000000000000000 ) ) ;
#15825=VECTOR ( 'NONE', #8505, 1000.000000000000000 ) ;
#15843=EDGE_LOOP ( 'NONE', ( #15062, #2581, #11531, #8333 ) ) ;
#15844=DIRECTION ( 'NONE',  ( -0.005931855436079598413, 0.9999824063907751803, 0.000000000000000000 ) ) ;
#15848=FACE_OUTER_BOUND ( 'NONE', #5771, .T. ) ;
#15855=DIRECTION ( 'NONE',  ( 0.000000000000000000, -1.000000000000000000, 0.000000000000000000 ) ) ;
#15874=ORIENTED_EDGE ( 'NONE', *, *, #5435, .F. ) ;
#15882=EDGE_CURVE ( 'NONE', #5376, #11530, #845, .T. ) ;
#15883=VECTOR ( 'NONE', #5399, 1000.000000000000000 ) ;
#15896=VERTEX_POINT ( 'NONE', #3349 ) ;
#15897=EDGE_LOOP ( 'NONE', ( #13208, #13207, #2396, #8079 ) ) ;
#15906=DIRECTION ( 'NONE',  ( 0.8660254037844410391, -0.4999999999999960032, -1.895741069380448091E-15 ) ) ;
#15932=CARTESIAN_POINT ( 'NONE',  ( -99.99999999999998579, -35.00000000000000711, 17.50000000000000000 ) ) ;
ENDSEC;
END-ISO-10303-21;
